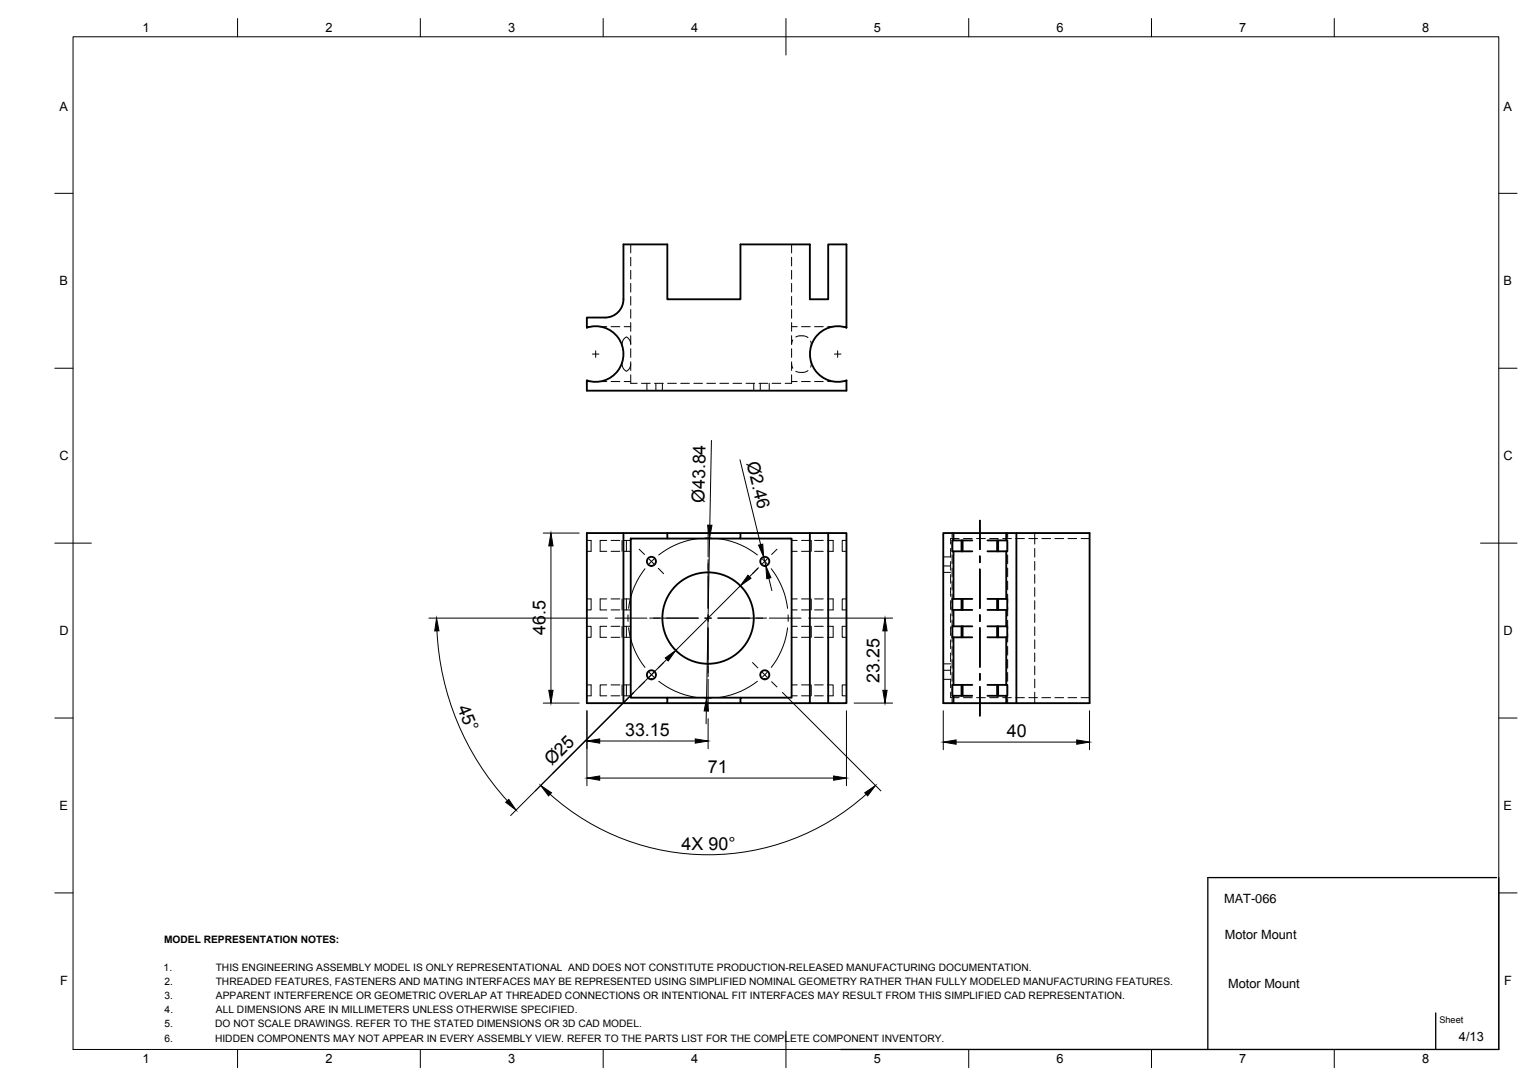
ISO-10303-21;
HEADER;
/* Generated by software containing ST-Developer
 * from STEP Tools, Inc. (www.steptools.com) 
 */

FILE_DESCRIPTION(
/* description */ ('CAx-IF Rec.Pracs.---Representation and Presentation of Product Manufa
cturing Information (PMI)---4.0---2014-10-13'),
/* implementation_level */ '2;1');

FILE_NAME(
/* name */ 'Motor Mount.step',
/* time_stamp */ '2026-10-24T15:58:00-07:00',
/* author */ (''),
/* organization */ (''),
/* preprocessor_version */ 'ST-DEVELOPER v20.2',
/* originating_system */ 'Autodesk Translation Framework v15.17.0.0',
/* authorisation */ '');

FILE_SCHEMA (('AP242_MANAGED_MODEL_BASED_3D_ENGINEERING_MIM_LF { 1 0 10303 442 2 1 4 }'));
ENDSEC;

DATA;
#10=MECHANICAL_DESIGN_GEOMETRIC_PRESENTATION_REPRESENTATION('',(#130),#8944);
#112=SHAPE_REPRESENTATION_RELATIONSHIP('SRR','None',#8994,#121);
#121=ADVANCED_BREP_SHAPE_REPRESENTATION('',(#139),#8935);
#130=STYLED_ITEM('',(#9053),#139);
#139=MANIFOLD_SOLID_BREP('Body1',#5151);
#165=CYLINDRICAL_SURFACE('',#5384,0.0125);
#166=CYLINDRICAL_SURFACE('',#5385,0.00123);
#167=CYLINDRICAL_SURFACE('',#5386,0.00123);
#168=CYLINDRICAL_SURFACE('',#5387,0.00123);
#169=CYLINDRICAL_SURFACE('',#5388,0.00123);
#170=CYLINDRICAL_SURFACE('',#5414,0.0076);
#171=CYLINDRICAL_SURFACE('',#5487,0.0023);
#172=CYLINDRICAL_SURFACE('',#5488,0.0023);
#173=CYLINDRICAL_SURFACE('',#5489,0.0023);
#174=CYLINDRICAL_SURFACE('',#5490,0.0023);
#175=CYLINDRICAL_SURFACE('',#5491,0.0023);
#176=CYLINDRICAL_SURFACE('',#5492,0.0023);
#177=CYLINDRICAL_SURFACE('',#5493,0.0023);
#178=CYLINDRICAL_SURFACE('',#5494,0.0023);
#179=CYLINDRICAL_SURFACE('',#5495,0.0023);
#180=CYLINDRICAL_SURFACE('',#5496,0.0023);
#181=CYLINDRICAL_SURFACE('',#5497,0.0023);
#182=CYLINDRICAL_SURFACE('',#5498,0.0023);
#183=CYLINDRICAL_SURFACE('',#5499,0.0023);
#184=CYLINDRICAL_SURFACE('',#5500,0.0023);
#185=CYLINDRICAL_SURFACE('',#5501,0.0023);
#186=CYLINDRICAL_SURFACE('',#5502,0.0023);
#187=CYLINDRICAL_SURFACE('',#5525,0.0076);
#188=CYLINDRICAL_SURFACE('',#5606,0.0023);
#189=CYLINDRICAL_SURFACE('',#5607,0.0023);
#190=CYLINDRICAL_SURFACE('',#5608,0.0023);
#191=CYLINDRICAL_SURFACE('',#5609,0.0023);
#192=CYLINDRICAL_SURFACE('',#5610,0.0023);
#193=CYLINDRICAL_SURFACE('',#5611,0.0023);
#194=CYLINDRICAL_SURFACE('',#5612,0.0023);
#195=CYLINDRICAL_SURFACE('',#5613,0.0023);
#196=CYLINDRICAL_SURFACE('',#5614,0.0023);
#197=CYLINDRICAL_SURFACE('',#5615,0.0023);
#198=CYLINDRICAL_SURFACE('',#5616,0.0023);
#199=CYLINDRICAL_SURFACE('',#5617,0.0023);
#200=CYLINDRICAL_SURFACE('',#5618,0.0023);
#201=CYLINDRICAL_SURFACE('',#5619,0.0023);
#202=CYLINDRICAL_SURFACE('',#5620,0.0023);
#203=CYLINDRICAL_SURFACE('',#5621,0.0023);
#204=CYLINDRICAL_SURFACE('',#5622,0.005);
#242=FACE_BOUND('',#613,.T.);
#243=FACE_BOUND('',#614,.T.);
#244=FACE_BOUND('',#615,.T.);
#245=FACE_BOUND('',#616,.T.);
#246=FACE_BOUND('',#617,.T.);
#247=FACE_BOUND('',#618,.T.);
#248=FACE_BOUND('',#619,.T.);
#249=FACE_BOUND('',#620,.T.);
#250=FACE_BOUND('',#634,.T.);
#251=FACE_BOUND('',#635,.T.);
#252=FACE_BOUND('',#636,.T.);
#253=FACE_BOUND('',#637,.T.);
#254=FACE_BOUND('',#638,.T.);
#255=FACE_BOUND('',#639,.T.);
#256=FACE_BOUND('',#640,.T.);
#257=FACE_BOUND('',#641,.T.);
#258=FACE_BOUND('',#659,.T.);
#259=FACE_BOUND('',#660,.T.);
#260=FACE_BOUND('',#661,.T.);
#261=FACE_BOUND('',#662,.T.);
#262=FACE_BOUND('',#663,.T.);
#263=FACE_BOUND('',#666,.T.);
#264=FACE_BOUND('',#667,.T.);
#265=FACE_BOUND('',#668,.T.);
#266=FACE_BOUND('',#669,.T.);
#267=FACE_BOUND('',#670,.T.);
#268=FACE_BOUND('',#694,.T.);
#269=FACE_BOUND('',#695,.T.);
#270=FACE_BOUND('',#696,.T.);
#271=FACE_BOUND('',#697,.T.);
#272=FACE_BOUND('',#698,.T.);
#273=FACE_BOUND('',#699,.T.);
#274=FACE_BOUND('',#700,.T.);
#275=FACE_BOUND('',#701,.T.);
#276=FACE_BOUND('',#758,.T.);
#277=FACE_BOUND('',#759,.T.);
#278=FACE_BOUND('',#760,.T.);
#279=FACE_BOUND('',#761,.T.);
#280=FACE_BOUND('',#762,.T.);
#281=FACE_BOUND('',#763,.T.);
#282=FACE_BOUND('',#764,.T.);
#283=FACE_BOUND('',#765,.T.);
#330=FACE_OUTER_BOUND('',#603,.T.);
#331=FACE_OUTER_BOUND('',#604,.T.);
#332=FACE_OUTER_BOUND('',#605,.T.);
#333=FACE_OUTER_BOUND('',#606,.T.);
#334=FACE_OUTER_BOUND('',#607,.T.);
#335=FACE_OUTER_BOUND('',#608,.T.);
#336=FACE_OUTER_BOUND('',#609,.T.);
#337=FACE_OUTER_BOUND('',#610,.T.);
#338=FACE_OUTER_BOUND('',#611,.T.);
#339=FACE_OUTER_BOUND('',#612,.T.);
#340=FACE_OUTER_BOUND('',#621,.T.);
#341=FACE_OUTER_BOUND('',#622,.T.);
#342=FACE_OUTER_BOUND('',#623,.T.);
#343=FACE_OUTER_BOUND('',#624,.T.);
#344=FACE_OUTER_BOUND('',#625,.T.);
#345=FACE_OUTER_BOUND('',#626,.T.);
#346=FACE_OUTER_BOUND('',#627,.T.);
#347=FACE_OUTER_BOUND('',#628,.T.);
#348=FACE_OUTER_BOUND('',#629,.T.);
#349=FACE_OUTER_BOUND('',#630,.T.);
#350=FACE_OUTER_BOUND('',#631,.T.);
#351=FACE_OUTER_BOUND('',#632,.T.);
#352=FACE_OUTER_BOUND('',#633,.T.);
#353=FACE_OUTER_BOUND('',#642,.T.);
#354=FACE_OUTER_BOUND('',#643,.T.);
#355=FACE_OUTER_BOUND('',#644,.T.);
#356=FACE_OUTER_BOUND('',#645,.T.);
#357=FACE_OUTER_BOUND('',#646,.T.);
#358=FACE_OUTER_BOUND('',#647,.T.);
#359=FACE_OUTER_BOUND('',#648,.T.);
#360=FACE_OUTER_BOUND('',#649,.T.);
#361=FACE_OUTER_BOUND('',#650,.T.);
#362=FACE_OUTER_BOUND('',#651,.T.);
#363=FACE_OUTER_BOUND('',#652,.T.);
#364=FACE_OUTER_BOUND('',#653,.T.);
#365=FACE_OUTER_BOUND('',#654,.T.);
#366=FACE_OUTER_BOUND('',#655,.T.);
#367=FACE_OUTER_BOUND('',#656,.T.);
#368=FACE_OUTER_BOUND('',#657,.T.);
#369=FACE_OUTER_BOUND('',#658,.T.);
#370=FACE_OUTER_BOUND('',#664,.T.);
#371=FACE_OUTER_BOUND('',#665,.T.);
#372=FACE_OUTER_BOUND('',#671,.T.);
#373=FACE_OUTER_BOUND('',#672,.T.);
#374=FACE_OUTER_BOUND('',#673,.T.);
#375=FACE_OUTER_BOUND('',#674,.T.);
#376=FACE_OUTER_BOUND('',#675,.T.);
#377=FACE_OUTER_BOUND('',#676,.T.);
#378=FACE_OUTER_BOUND('',#677,.T.);
#379=FACE_OUTER_BOUND('',#678,.T.);
#380=FACE_OUTER_BOUND('',#679,.T.);
#381=FACE_OUTER_BOUND('',#680,.T.);
#382=FACE_OUTER_BOUND('',#681,.T.);
#383=FACE_OUTER_BOUND('',#682,.T.);
#384=FACE_OUTER_BOUND('',#683,.T.);
#385=FACE_OUTER_BOUND('',#684,.T.);
#386=FACE_OUTER_BOUND('',#685,.T.);
#387=FACE_OUTER_BOUND('',#686,.T.);
#388=FACE_OUTER_BOUND('',#687,.T.);
#389=FACE_OUTER_BOUND('',#688,.T.);
#390=FACE_OUTER_BOUND('',#689,.T.);
#391=FACE_OUTER_BOUND('',#690,.T.);
#392=FACE_OUTER_BOUND('',#691,.T.);
#393=FACE_OUTER_BOUND('',#692,.T.);
#394=FACE_OUTER_BOUND('',#693,.T.);
#395=FACE_OUTER_BOUND('',#702,.T.);
#396=FACE_OUTER_BOUND('',#703,.T.);
#397=FACE_OUTER_BOUND('',#704,.T.);
#398=FACE_OUTER_BOUND('',#705,.T.);
#399=FACE_OUTER_BOUND('',#706,.T.);
#400=FACE_OUTER_BOUND('',#707,.T.);
#401=FACE_OUTER_BOUND('',#708,.T.);
#402=FACE_OUTER_BOUND('',#709,.T.);
#403=FACE_OUTER_BOUND('',#710,.T.);
#404=FACE_OUTER_BOUND('',#711,.T.);
#405=FACE_OUTER_BOUND('',#712,.T.);
#406=FACE_OUTER_BOUND('',#713,.T.);
#407=FACE_OUTER_BOUND('',#714,.T.);
#408=FACE_OUTER_BOUND('',#715,.T.);
#409=FACE_OUTER_BOUND('',#716,.T.);
#410=FACE_OUTER_BOUND('',#717,.T.);
#411=FACE_OUTER_BOUND('',#718,.T.);
#412=FACE_OUTER_BOUND('',#719,.T.);
#413=FACE_OUTER_BOUND('',#720,.T.);
#414=FACE_OUTER_BOUND('',#721,.T.);
#415=FACE_OUTER_BOUND('',#722,.T.);
#416=FACE_OUTER_BOUND('',#723,.T.);
#417=FACE_OUTER_BOUND('',#724,.T.);
#418=FACE_OUTER_BOUND('',#725,.T.);
#419=FACE_OUTER_BOUND('',#726,.T.);
#420=FACE_OUTER_BOUND('',#727,.T.);
#421=FACE_OUTER_BOUND('',#728,.T.);
#422=FACE_OUTER_BOUND('',#729,.T.);
#423=FACE_OUTER_BOUND('',#730,.T.);
#424=FACE_OUTER_BOUND('',#731,.T.);
#425=FACE_OUTER_BOUND('',#732,.T.);
#426=FACE_OUTER_BOUND('',#733,.T.);
#427=FACE_OUTER_BOUND('',#734,.T.);
#428=FACE_OUTER_BOUND('',#735,.T.);
#429=FACE_OUTER_BOUND('',#736,.T.);
#430=FACE_OUTER_BOUND('',#737,.T.);
#431=FACE_OUTER_BOUND('',#738,.T.);
#432=FACE_OUTER_BOUND('',#739,.T.);
#433=FACE_OUTER_BOUND('',#740,.T.);
#434=FACE_OUTER_BOUND('',#741,.T.);
#435=FACE_OUTER_BOUND('',#742,.T.);
#436=FACE_OUTER_BOUND('',#743,.T.);
#437=FACE_OUTER_BOUND('',#744,.T.);
#438=FACE_OUTER_BOUND('',#745,.T.);
#439=FACE_OUTER_BOUND('',#746,.T.);
#440=FACE_OUTER_BOUND('',#747,.T.);
#441=FACE_OUTER_BOUND('',#748,.T.);
#442=FACE_OUTER_BOUND('',#749,.T.);
#443=FACE_OUTER_BOUND('',#750,.T.);
#444=FACE_OUTER_BOUND('',#751,.T.);
#445=FACE_OUTER_BOUND('',#752,.T.);
#446=FACE_OUTER_BOUND('',#753,.T.);
#447=FACE_OUTER_BOUND('',#754,.T.);
#448=FACE_OUTER_BOUND('',#755,.T.);
#449=FACE_OUTER_BOUND('',#756,.T.);
#450=FACE_OUTER_BOUND('',#757,.T.);
#451=FACE_OUTER_BOUND('',#766,.T.);
#452=FACE_OUTER_BOUND('',#767,.T.);
#453=FACE_OUTER_BOUND('',#768,.T.);
#454=FACE_OUTER_BOUND('',#769,.T.);
#455=FACE_OUTER_BOUND('',#770,.T.);
#456=FACE_OUTER_BOUND('',#771,.T.);
#457=FACE_OUTER_BOUND('',#772,.T.);
#458=FACE_OUTER_BOUND('',#773,.T.);
#459=FACE_OUTER_BOUND('',#774,.T.);
#460=FACE_OUTER_BOUND('',#775,.T.);
#461=FACE_OUTER_BOUND('',#776,.T.);
#462=FACE_OUTER_BOUND('',#777,.T.);
#463=FACE_OUTER_BOUND('',#778,.T.);
#464=FACE_OUTER_BOUND('',#779,.T.);
#465=FACE_OUTER_BOUND('',#780,.T.);
#466=FACE_OUTER_BOUND('',#781,.T.);
#467=FACE_OUTER_BOUND('',#782,.T.);
#468=FACE_OUTER_BOUND('',#783,.T.);
#469=FACE_OUTER_BOUND('',#784,.T.);
#470=FACE_OUTER_BOUND('',#785,.T.);
#471=FACE_OUTER_BOUND('',#786,.T.);
#472=FACE_OUTER_BOUND('',#787,.T.);
#473=FACE_OUTER_BOUND('',#788,.T.);
#474=FACE_OUTER_BOUND('',#789,.T.);
#475=FACE_OUTER_BOUND('',#790,.T.);
#476=FACE_OUTER_BOUND('',#791,.T.);
#477=FACE_OUTER_BOUND('',#792,.T.);
#478=FACE_OUTER_BOUND('',#793,.T.);
#479=FACE_OUTER_BOUND('',#794,.T.);
#480=FACE_OUTER_BOUND('',#795,.T.);
#481=FACE_OUTER_BOUND('',#796,.T.);
#482=FACE_OUTER_BOUND('',#797,.T.);
#483=FACE_OUTER_BOUND('',#798,.T.);
#484=FACE_OUTER_BOUND('',#799,.T.);
#485=FACE_OUTER_BOUND('',#800,.T.);
#486=FACE_OUTER_BOUND('',#801,.T.);
#487=FACE_OUTER_BOUND('',#802,.T.);
#488=FACE_OUTER_BOUND('',#803,.T.);
#489=FACE_OUTER_BOUND('',#804,.T.);
#490=FACE_OUTER_BOUND('',#805,.T.);
#491=FACE_OUTER_BOUND('',#806,.T.);
#492=FACE_OUTER_BOUND('',#807,.T.);
#493=FACE_OUTER_BOUND('',#808,.T.);
#494=FACE_OUTER_BOUND('',#809,.T.);
#495=FACE_OUTER_BOUND('',#810,.T.);
#496=FACE_OUTER_BOUND('',#811,.T.);
#497=FACE_OUTER_BOUND('',#812,.T.);
#498=FACE_OUTER_BOUND('',#813,.T.);
#499=FACE_OUTER_BOUND('',#814,.T.);
#603=EDGE_LOOP('',(#3395,#3396,#3397,#3398));
#604=EDGE_LOOP('',(#3399,#3400,#3401,#3402));
#605=EDGE_LOOP('',(#3403,#3404,#3405,#3406));
#606=EDGE_LOOP('',(#3407,#3408,#3409,#3410,#3411,#3412,#3413,#3414));
#607=EDGE_LOOP('',(#3415,#3416,#3417,#3418,#3419,#3420,#3421,#3422));
#608=EDGE_LOOP('',(#3423,#3424,#3425,#3426,#3427,#3428,#3429,#3430));
#609=EDGE_LOOP('',(#3431,#3432,#3433,#3434));
#610=EDGE_LOOP('',(#3435,#3436,#3437,#3438));
#611=EDGE_LOOP('',(#3439,#3440,#3441,#3442));
#612=EDGE_LOOP('',(#3443,#3444,#3445,#3446));
#613=EDGE_LOOP('',(#3447,#3448,#3449,#3450));
#614=EDGE_LOOP('',(#3451,#3452,#3453,#3454));
#615=EDGE_LOOP('',(#3455,#3456,#3457,#3458));
#616=EDGE_LOOP('',(#3459,#3460,#3461,#3462));
#617=EDGE_LOOP('',(#3463,#3464,#3465,#3466));
#618=EDGE_LOOP('',(#3467,#3468,#3469,#3470));
#619=EDGE_LOOP('',(#3471,#3472,#3473,#3474));
#620=EDGE_LOOP('',(#3475,#3476,#3477,#3478));
#621=EDGE_LOOP('',(#3479,#3480,#3481));
#622=EDGE_LOOP('',(#3482,#3483,#3484));
#623=EDGE_LOOP('',(#3485,#3486,#3487));
#624=EDGE_LOOP('',(#3488,#3489,#3490));
#625=EDGE_LOOP('',(#3491,#3492,#3493));
#626=EDGE_LOOP('',(#3494,#3495,#3496));
#627=EDGE_LOOP('',(#3497,#3498,#3499,#3500));
#628=EDGE_LOOP('',(#3501,#3502,#3503));
#629=EDGE_LOOP('',(#3504,#3505,#3506));
#630=EDGE_LOOP('',(#3507,#3508,#3509));
#631=EDGE_LOOP('',(#3510,#3511,#3512,#3513,#3514,#3515,#3516,#3517,#3518,
#3519,#3520,#3521,#3522,#3523,#3524,#3525,#3526,#3527,#3528,#3529));
#632=EDGE_LOOP('',(#3530,#3531,#3532,#3533));
#633=EDGE_LOOP('',(#3534,#3535,#3536,#3537));
#634=EDGE_LOOP('',(#3538,#3539,#3540,#3541));
#635=EDGE_LOOP('',(#3542,#3543,#3544,#3545));
#636=EDGE_LOOP('',(#3546,#3547,#3548,#3549));
#637=EDGE_LOOP('',(#3550,#3551,#3552,#3553));
#638=EDGE_LOOP('',(#3554,#3555,#3556,#3557));
#639=EDGE_LOOP('',(#3558,#3559,#3560,#3561));
#640=EDGE_LOOP('',(#3562,#3563,#3564,#3565));
#641=EDGE_LOOP('',(#3566,#3567,#3568,#3569));
#642=EDGE_LOOP('',(#3570,#3571,#3572));
#643=EDGE_LOOP('',(#3573,#3574,#3575));
#644=EDGE_LOOP('',(#3576,#3577,#3578));
#645=EDGE_LOOP('',(#3579,#3580,#3581,#3582));
#646=EDGE_LOOP('',(#3583,#3584,#3585,#3586));
#647=EDGE_LOOP('',(#3587,#3588,#3589,#3590));
#648=EDGE_LOOP('',(#3591,#3592,#3593));
#649=EDGE_LOOP('',(#3594,#3595,#3596));
#650=EDGE_LOOP('',(#3597,#3598,#3599,#3600));
#651=EDGE_LOOP('',(#3601,#3602,#3603,#3604));
#652=EDGE_LOOP('',(#3605,#3606,#3607,#3608));
#653=EDGE_LOOP('',(#3609,#3610,#3611,#3612));
#654=EDGE_LOOP('',(#3613,#3614,#3615,#3616,#3617,#3618,#3619,#3620,#3621,
#3622,#3623,#3624,#3625,#3626,#3627,#3628,#3629,#3630,#3631,#3632));
#655=EDGE_LOOP('',(#3633,#3634,#3635,#3636));
#656=EDGE_LOOP('',(#3637,#3638,#3639,#3640,#3641,#3642,#3643,#3644));
#657=EDGE_LOOP('',(#3645,#3646,#3647,#3648,#3649,#3650,#3651,#3652,#3653,
#3654,#3655,#3656,#3657,#3658,#3659,#3660,#3661,#3662,#3663));
#658=EDGE_LOOP('',(#3664,#3665,#3666,#3667));
#659=EDGE_LOOP('',(#3668));
#660=EDGE_LOOP('',(#3669));
#661=EDGE_LOOP('',(#3670));
#662=EDGE_LOOP('',(#3671));
#663=EDGE_LOOP('',(#3672));
#664=EDGE_LOOP('',(#3673,#3674,#3675,#3676,#3677,#3678,#3679,#3680,#3681,
#3682,#3683,#3684,#3685,#3686,#3687,#3688,#3689,#3690,#3691));
#665=EDGE_LOOP('',(#3692,#3693,#3694,#3695));
#666=EDGE_LOOP('',(#3696));
#667=EDGE_LOOP('',(#3697));
#668=EDGE_LOOP('',(#3698));
#669=EDGE_LOOP('',(#3699));
#670=EDGE_LOOP('',(#3700));
#671=EDGE_LOOP('',(#3701,#3702,#3703,#3704));
#672=EDGE_LOOP('',(#3705,#3706,#3707,#3708));
#673=EDGE_LOOP('',(#3709,#3710,#3711,#3712));
#674=EDGE_LOOP('',(#3713,#3714,#3715,#3716));
#675=EDGE_LOOP('',(#3717,#3718,#3719,#3720));
#676=EDGE_LOOP('',(#3721,#3722,#3723,#3724));
#677=EDGE_LOOP('',(#3725,#3726,#3727,#3728));
#678=EDGE_LOOP('',(#3729,#3730,#3731,#3732));
#679=EDGE_LOOP('',(#3733,#3734,#3735,#3736));
#680=EDGE_LOOP('',(#3737,#3738,#3739));
#681=EDGE_LOOP('',(#3740,#3741,#3742));
#682=EDGE_LOOP('',(#3743,#3744,#3745));
#683=EDGE_LOOP('',(#3746,#3747,#3748));
#684=EDGE_LOOP('',(#3749,#3750,#3751));
#685=EDGE_LOOP('',(#3752,#3753,#3754));
#686=EDGE_LOOP('',(#3755,#3756,#3757,#3758));
#687=EDGE_LOOP('',(#3759,#3760,#3761));
#688=EDGE_LOOP('',(#3762,#3763,#3764));
#689=EDGE_LOOP('',(#3765,#3766,#3767));
#690=EDGE_LOOP('',(#3768,#3769,#3770));
#691=EDGE_LOOP('',(#3771,#3772,#3773));
#692=EDGE_LOOP('',(#3774,#3775,#3776,#3777,#3778,#3779,#3780,#3781,#3782,
#3783,#3784,#3785,#3786,#3787,#3788,#3789,#3790,#3791,#3792,#3793));
#693=EDGE_LOOP('',(#3794,#3795,#3796,#3797,#3798,#3799,#3800,#3801,#3802,
#3803,#3804,#3805,#3806,#3807,#3808,#3809,#3810,#3811,#3812,#3813,#3814,
#3815,#3816,#3817,#3818,#3819,#3820,#3821,#3822,#3823,#3824,#3825,#3826,
#3827,#3828,#3829));
#694=EDGE_LOOP('',(#3830,#3831,#3832,#3833));
#695=EDGE_LOOP('',(#3834,#3835,#3836,#3837));
#696=EDGE_LOOP('',(#3838,#3839,#3840,#3841));
#697=EDGE_LOOP('',(#3842,#3843,#3844,#3845));
#698=EDGE_LOOP('',(#3846,#3847,#3848,#3849));
#699=EDGE_LOOP('',(#3850,#3851,#3852,#3853));
#700=EDGE_LOOP('',(#3854,#3855,#3856,#3857));
#701=EDGE_LOOP('',(#3858,#3859,#3860,#3861));
#702=EDGE_LOOP('',(#3862,#3863,#3864,#3865,#3866));
#703=EDGE_LOOP('',(#3867,#3868,#3869,#3870));
#704=EDGE_LOOP('',(#3871,#3872,#3873,#3874,#3875));
#705=EDGE_LOOP('',(#3876,#3877,#3878,#3879));
#706=EDGE_LOOP('',(#3880,#3881,#3882,#3883,#3884));
#707=EDGE_LOOP('',(#3885,#3886,#3887,#3888,#3889));
#708=EDGE_LOOP('',(#3890,#3891,#3892,#3893,#3894));
#709=EDGE_LOOP('',(#3895,#3896,#3897,#3898));
#710=EDGE_LOOP('',(#3899,#3900,#3901,#3902,#3903));
#711=EDGE_LOOP('',(#3904,#3905,#3906,#3907,#3908));
#712=EDGE_LOOP('',(#3909,#3910,#3911,#3912));
#713=EDGE_LOOP('',(#3913,#3914,#3915,#3916,#3917));
#714=EDGE_LOOP('',(#3918,#3919,#3920,#3921,#3922));
#715=EDGE_LOOP('',(#3923,#3924,#3925,#3926));
#716=EDGE_LOOP('',(#3927,#3928,#3929,#3930,#3931));
#717=EDGE_LOOP('',(#3932,#3933,#3934,#3935,#3936));
#718=EDGE_LOOP('',(#3937,#3938,#3939,#3940));
#719=EDGE_LOOP('',(#3941,#3942,#3943,#3944,#3945));
#720=EDGE_LOOP('',(#3946,#3947,#3948,#3949));
#721=EDGE_LOOP('',(#3950,#3951,#3952,#3953,#3954));
#722=EDGE_LOOP('',(#3955,#3956,#3957,#3958,#3959));
#723=EDGE_LOOP('',(#3960,#3961,#3962,#3963));
#724=EDGE_LOOP('',(#3964,#3965,#3966,#3967,#3968));
#725=EDGE_LOOP('',(#3969,#3970,#3971,#3972,#3973));
#726=EDGE_LOOP('',(#3974,#3975,#3976,#3977));
#727=EDGE_LOOP('',(#3978,#3979,#3980,#3981));
#728=EDGE_LOOP('',(#3982,#3983,#3984,#3985));
#729=EDGE_LOOP('',(#3986,#3987,#3988,#3989));
#730=EDGE_LOOP('',(#3990,#3991,#3992,#3993));
#731=EDGE_LOOP('',(#3994,#3995,#3996,#3997));
#732=EDGE_LOOP('',(#3998,#3999,#4000,#4001));
#733=EDGE_LOOP('',(#4002,#4003,#4004,#4005));
#734=EDGE_LOOP('',(#4006,#4007,#4008,#4009));
#735=EDGE_LOOP('',(#4010,#4011,#4012,#4013));
#736=EDGE_LOOP('',(#4014,#4015,#4016,#4017));
#737=EDGE_LOOP('',(#4018,#4019,#4020,#4021));
#738=EDGE_LOOP('',(#4022,#4023,#4024,#4025));
#739=EDGE_LOOP('',(#4026,#4027,#4028,#4029));
#740=EDGE_LOOP('',(#4030,#4031,#4032,#4033));
#741=EDGE_LOOP('',(#4034,#4035,#4036,#4037));
#742=EDGE_LOOP('',(#4038,#4039,#4040));
#743=EDGE_LOOP('',(#4041,#4042,#4043,#4044));
#744=EDGE_LOOP('',(#4045,#4046,#4047));
#745=EDGE_LOOP('',(#4048,#4049,#4050,#4051));
#746=EDGE_LOOP('',(#4052,#4053,#4054));
#747=EDGE_LOOP('',(#4055,#4056,#4057));
#748=EDGE_LOOP('',(#4058,#4059,#4060));
#749=EDGE_LOOP('',(#4061,#4062,#4063,#4064));
#750=EDGE_LOOP('',(#4065,#4066,#4067));
#751=EDGE_LOOP('',(#4068,#4069,#4070,#4071));
#752=EDGE_LOOP('',(#4072,#4073,#4074));
#753=EDGE_LOOP('',(#4075,#4076,#4077,#4078));
#754=EDGE_LOOP('',(#4079,#4080,#4081,#4082));
#755=EDGE_LOOP('',(#4083,#4084,#4085,#4086));
#756=EDGE_LOOP('',(#4087,#4088,#4089,#4090,#4091,#4092,#4093,#4094,#4095,
#4096,#4097,#4098,#4099,#4100,#4101,#4102,#4103,#4104,#4105,#4106));
#757=EDGE_LOOP('',(#4107,#4108,#4109,#4110,#4111,#4112,#4113,#4114,#4115,
#4116,#4117,#4118,#4119,#4120,#4121,#4122,#4123,#4124,#4125,#4126,#4127,
#4128,#4129,#4130,#4131,#4132,#4133,#4134,#4135,#4136,#4137,#4138,#4139,
#4140,#4141,#4142));
#758=EDGE_LOOP('',(#4143,#4144,#4145,#4146));
#759=EDGE_LOOP('',(#4147,#4148,#4149,#4150));
#760=EDGE_LOOP('',(#4151,#4152,#4153,#4154));
#761=EDGE_LOOP('',(#4155,#4156,#4157,#4158));
#762=EDGE_LOOP('',(#4159,#4160,#4161,#4162));
#763=EDGE_LOOP('',(#4163,#4164,#4165,#4166));
#764=EDGE_LOOP('',(#4167,#4168,#4169,#4170));
#765=EDGE_LOOP('',(#4171,#4172,#4173,#4174));
#766=EDGE_LOOP('',(#4175,#4176,#4177,#4178));
#767=EDGE_LOOP('',(#4179,#4180,#4181,#4182,#4183,#4184));
#768=EDGE_LOOP('',(#4185,#4186,#4187,#4188));
#769=EDGE_LOOP('',(#4189,#4190,#4191,#4192,#4193,#4194));
#770=EDGE_LOOP('',(#4195,#4196,#4197,#4198));
#771=EDGE_LOOP('',(#4199,#4200,#4201,#4202,#4203,#4204));
#772=EDGE_LOOP('',(#4205,#4206,#4207,#4208));
#773=EDGE_LOOP('',(#4209,#4210,#4211,#4212,#4213,#4214));
#774=EDGE_LOOP('',(#4215,#4216,#4217,#4218));
#775=EDGE_LOOP('',(#4219,#4220,#4221,#4222,#4223,#4224));
#776=EDGE_LOOP('',(#4225,#4226,#4227,#4228));
#777=EDGE_LOOP('',(#4229,#4230,#4231,#4232,#4233,#4234));
#778=EDGE_LOOP('',(#4235,#4236,#4237,#4238));
#779=EDGE_LOOP('',(#4239,#4240,#4241,#4242,#4243,#4244));
#780=EDGE_LOOP('',(#4245,#4246,#4247,#4248));
#781=EDGE_LOOP('',(#4249,#4250,#4251,#4252,#4253,#4254));
#782=EDGE_LOOP('',(#4255,#4256,#4257,#4258));
#783=EDGE_LOOP('',(#4259,#4260,#4261,#4262,#4263,#4264));
#784=EDGE_LOOP('',(#4265,#4266,#4267,#4268));
#785=EDGE_LOOP('',(#4269,#4270,#4271,#4272,#4273,#4274));
#786=EDGE_LOOP('',(#4275,#4276,#4277,#4278));
#787=EDGE_LOOP('',(#4279,#4280,#4281,#4282,#4283,#4284));
#788=EDGE_LOOP('',(#4285,#4286,#4287,#4288));
#789=EDGE_LOOP('',(#4289,#4290,#4291,#4292,#4293,#4294));
#790=EDGE_LOOP('',(#4295,#4296,#4297,#4298));
#791=EDGE_LOOP('',(#4299,#4300,#4301,#4302,#4303,#4304));
#792=EDGE_LOOP('',(#4305,#4306,#4307,#4308));
#793=EDGE_LOOP('',(#4309,#4310,#4311,#4312,#4313,#4314));
#794=EDGE_LOOP('',(#4315,#4316,#4317,#4318));
#795=EDGE_LOOP('',(#4319,#4320,#4321,#4322,#4323,#4324));
#796=EDGE_LOOP('',(#4325,#4326,#4327,#4328));
#797=EDGE_LOOP('',(#4329,#4330,#4331,#4332,#4333,#4334));
#798=EDGE_LOOP('',(#4335,#4336,#4337,#4338));
#799=EDGE_LOOP('',(#4339,#4340,#4341,#4342));
#800=EDGE_LOOP('',(#4343,#4344,#4345,#4346));
#801=EDGE_LOOP('',(#4347,#4348,#4349,#4350));
#802=EDGE_LOOP('',(#4351,#4352,#4353,#4354));
#803=EDGE_LOOP('',(#4355,#4356,#4357,#4358));
#804=EDGE_LOOP('',(#4359,#4360,#4361,#4362));
#805=EDGE_LOOP('',(#4363,#4364,#4365,#4366));
#806=EDGE_LOOP('',(#4367,#4368,#4369,#4370));
#807=EDGE_LOOP('',(#4371,#4372,#4373,#4374));
#808=EDGE_LOOP('',(#4375,#4376,#4377,#4378));
#809=EDGE_LOOP('',(#4379,#4380,#4381,#4382));
#810=EDGE_LOOP('',(#4383,#4384,#4385,#4386));
#811=EDGE_LOOP('',(#4387,#4388,#4389,#4390));
#812=EDGE_LOOP('',(#4391,#4392,#4393,#4394));
#813=EDGE_LOOP('',(#4395,#4396,#4397,#4398));
#814=EDGE_LOOP('',(#4399,#4400,#4401,#4402));
#941=CIRCLE('',#5320,0.0076);
#942=CIRCLE('',#5322,0.0076);
#943=CIRCLE('',#5324,0.0076);
#944=CIRCLE('',#5326,0.0076);
#945=CIRCLE('',#5328,0.0076);
#946=CIRCLE('',#5330,0.0076);
#947=CIRCLE('',#5333,0.0076);
#948=CIRCLE('',#5335,0.0076);
#949=CIRCLE('',#5337,0.0076);
#950=CIRCLE('',#5342,0.0076);
#951=CIRCLE('',#5344,0.0076);
#952=CIRCLE('',#5346,0.0076);
#953=CIRCLE('',#5351,0.0076);
#954=CIRCLE('',#5353,0.0076);
#955=CIRCLE('',#5362,0.0076);
#956=CIRCLE('',#5363,0.005);
#957=CIRCLE('',#5364,0.0076);
#958=CIRCLE('',#5366,0.00123);
#959=CIRCLE('',#5367,0.00123);
#960=CIRCLE('',#5368,0.00123);
#961=CIRCLE('',#5369,0.00123);
#962=CIRCLE('',#5370,0.0125);
#963=CIRCLE('',#5372,0.0076);
#964=CIRCLE('',#5373,0.0076);
#965=CIRCLE('',#5374,0.005);
#966=CIRCLE('',#5376,0.00123);
#967=CIRCLE('',#5377,0.00123);
#968=CIRCLE('',#5378,0.00123);
#969=CIRCLE('',#5379,0.00123);
#970=CIRCLE('',#5380,0.0125);
#971=CIRCLE('',#5391,0.0076);
#972=CIRCLE('',#5393,0.0076);
#973=CIRCLE('',#5395,0.0076);
#974=CIRCLE('',#5397,0.0076);
#975=CIRCLE('',#5399,0.0076);
#976=CIRCLE('',#5401,0.0076);
#977=CIRCLE('',#5404,0.0076);
#978=CIRCLE('',#5406,0.0076);
#979=CIRCLE('',#5408,0.0076);
#980=CIRCLE('',#5410,0.0076);
#981=CIRCLE('',#5412,0.0076);
#982=CIRCLE('',#5415,0.0076);
#983=CIRCLE('',#5416,0.0076);
#984=CIRCLE('',#5417,0.0076);
#985=CIRCLE('',#5418,0.0076);
#986=CIRCLE('',#5419,0.0076);
#987=CIRCLE('',#5420,0.0076);
#988=CIRCLE('',#5421,0.0076);
#989=CIRCLE('',#5422,0.0076);
#990=CIRCLE('',#5423,0.0076);
#991=CIRCLE('',#5424,0.0076);
#992=CIRCLE('',#5425,0.0076);
#993=CIRCLE('',#5426,0.0076);
#994=CIRCLE('',#5427,0.0076);
#995=CIRCLE('',#5428,0.0076);
#996=CIRCLE('',#5429,0.0076);
#997=CIRCLE('',#5430,0.0076);
#998=CIRCLE('',#5432,0.0023);
#999=CIRCLE('',#5433,0.0023);
#1000=CIRCLE('',#5436,0.0023);
#1001=CIRCLE('',#5437,0.0023);
#1002=CIRCLE('',#5440,0.0023);
#1003=CIRCLE('',#5441,0.0023);
#1004=CIRCLE('',#5443,0.0023);
#1005=CIRCLE('',#5444,0.0023);
#1006=CIRCLE('',#5446,0.0023);
#1007=CIRCLE('',#5447,0.0023);
#1008=CIRCLE('',#5450,0.0023);
#1009=CIRCLE('',#5451,0.0023);
#1010=CIRCLE('',#5453,0.0023);
#1011=CIRCLE('',#5454,0.0023);
#1012=CIRCLE('',#5457,0.0023);
#1013=CIRCLE('',#5458,0.0023);
#1014=CIRCLE('',#5460,0.0023);
#1015=CIRCLE('',#5461,0.0023);
#1016=CIRCLE('',#5464,0.0023);
#1017=CIRCLE('',#5465,0.0023);
#1018=CIRCLE('',#5467,0.0023);
#1019=CIRCLE('',#5468,0.0023);
#1020=CIRCLE('',#5471,0.0023);
#1021=CIRCLE('',#5472,0.0023);
#1022=CIRCLE('',#5475,0.0023);
#1023=CIRCLE('',#5476,0.0023);
#1024=CIRCLE('',#5478,0.0023);
#1025=CIRCLE('',#5479,0.0023);
#1026=CIRCLE('',#5482,0.0023);
#1027=CIRCLE('',#5483,0.0023);
#1028=CIRCLE('',#5485,0.0023);
#1029=CIRCLE('',#5486,0.0023);
#1030=CIRCLE('',#5504,0.0076);
#1031=CIRCLE('',#5507,0.0076);
#1032=CIRCLE('',#5510,0.0076);
#1033=CIRCLE('',#5512,0.0076);
#1034=CIRCLE('',#5514,0.0076);
#1035=CIRCLE('',#5517,0.0076);
#1036=CIRCLE('',#5520,0.0076);
#1037=CIRCLE('',#5526,0.0076);
#1038=CIRCLE('',#5527,0.0076);
#1039=CIRCLE('',#5528,0.0076);
#1040=CIRCLE('',#5529,0.0076);
#1041=CIRCLE('',#5530,0.0076);
#1042=CIRCLE('',#5531,0.0076);
#1043=CIRCLE('',#5532,0.0076);
#1044=CIRCLE('',#5533,0.0076);
#1045=CIRCLE('',#5534,0.0076);
#1046=CIRCLE('',#5535,0.0076);
#1047=CIRCLE('',#5536,0.0076);
#1048=CIRCLE('',#5537,0.0076);
#1049=CIRCLE('',#5538,0.0076);
#1050=CIRCLE('',#5539,0.0076);
#1051=CIRCLE('',#5540,0.0076);
#1052=CIRCLE('',#5541,0.0076);
#1053=CIRCLE('',#5544,0.0023);
#1054=CIRCLE('',#5545,0.0023);
#1055=CIRCLE('',#5548,0.0023);
#1056=CIRCLE('',#5549,0.0023);
#1057=CIRCLE('',#5552,0.0023);
#1058=CIRCLE('',#5553,0.0023);
#1059=CIRCLE('',#5556,0.0023);
#1060=CIRCLE('',#5557,0.0023);
#1061=CIRCLE('',#5560,0.0023);
#1062=CIRCLE('',#5561,0.0023);
#1063=CIRCLE('',#5564,0.0023);
#1064=CIRCLE('',#5565,0.0023);
#1065=CIRCLE('',#5568,0.0023);
#1066=CIRCLE('',#5569,0.0023);
#1067=CIRCLE('',#5572,0.0023);
#1068=CIRCLE('',#5573,0.0023);
#1069=CIRCLE('',#5576,0.0023);
#1070=CIRCLE('',#5577,0.0023);
#1071=CIRCLE('',#5580,0.0023);
#1072=CIRCLE('',#5581,0.0023);
#1073=CIRCLE('',#5584,0.0023);
#1074=CIRCLE('',#5585,0.0023);
#1075=CIRCLE('',#5588,0.0023);
#1076=CIRCLE('',#5589,0.0023);
#1077=CIRCLE('',#5592,0.0023);
#1078=CIRCLE('',#5593,0.0023);
#1079=CIRCLE('',#5596,0.0023);
#1080=CIRCLE('',#5597,0.0023);
#1081=CIRCLE('',#5600,0.0023);
#1082=CIRCLE('',#5601,0.0023);
#1083=CIRCLE('',#5604,0.0023);
#1084=CIRCLE('',#5605,0.0023);
#1204=LINE('',#7535,#1659);
#1205=LINE('',#7537,#1660);
#1206=LINE('',#7539,#1661);
#1207=LINE('',#7540,#1662);
#1208=LINE('',#7544,#1663);
#1209=LINE('',#7546,#1664);
#1210=LINE('',#7548,#1665);
#1211=LINE('',#7549,#1666);
#1212=LINE('',#7551,#1667);
#1213=LINE('',#7552,#1668);
#1214=LINE('',#7555,#1669);
#1215=LINE('',#7557,#1670);
#1216=LINE('',#7559,#1671);
#1217=LINE('',#7561,#1672);
#1218=LINE('',#7563,#1673);
#1219=LINE('',#7565,#1674);
#1220=LINE('',#7566,#1675);
#1221=LINE('',#7569,#1676);
#1222=LINE('',#7571,#1677);
#1223=LINE('',#7573,#1678);
#1224=LINE('',#7575,#1679);
#1225=LINE('',#7577,#1680);
#1226=LINE('',#7579,#1681);
#1227=LINE('',#7580,#1682);
#1228=LINE('',#7583,#1683);
#1229=LINE('',#7585,#1684);
#1230=LINE('',#7586,#1685);
#1231=LINE('',#7590,#1686);
#1232=LINE('',#7592,#1687);
#1233=LINE('',#7594,#1688);
#1234=LINE('',#7595,#1689);
#1235=LINE('',#7598,#1690);
#1236=LINE('',#7600,#1691);
#1237=LINE('',#7601,#1692);
#1238=LINE('',#7605,#1693);
#1239=LINE('',#7606,#1694);
#1240=LINE('',#7607,#1695);
#1241=LINE('',#7610,#1696);
#1242=LINE('',#7611,#1697);
#1243=LINE('',#7614,#1698);
#1244=LINE('',#7616,#1699);
#1245=LINE('',#7618,#1700);
#1246=LINE('',#7619,#1701);
#1247=LINE('',#7622,#1702);
#1248=LINE('',#7624,#1703);
#1249=LINE('',#7626,#1704);
#1250=LINE('',#7627,#1705);
#1251=LINE('',#7630,#1706);
#1252=LINE('',#7632,#1707);
#1253=LINE('',#7634,#1708);
#1254=LINE('',#7635,#1709);
#1255=LINE('',#7638,#1710);
#1256=LINE('',#7640,#1711);
#1257=LINE('',#7642,#1712);
#1258=LINE('',#7643,#1713);
#1259=LINE('',#7646,#1714);
#1260=LINE('',#7648,#1715);
#1261=LINE('',#7650,#1716);
#1262=LINE('',#7651,#1717);
#1263=LINE('',#7654,#1718);
#1264=LINE('',#7656,#1719);
#1265=LINE('',#7658,#1720);
#1266=LINE('',#7659,#1721);
#1267=LINE('',#7662,#1722);
#1268=LINE('',#7664,#1723);
#1269=LINE('',#7666,#1724);
#1270=LINE('',#7667,#1725);
#1271=LINE('',#7670,#1726);
#1272=LINE('',#7672,#1727);
#1273=LINE('',#7674,#1728);
#1274=LINE('',#7675,#1729);
#1275=LINE('',#7681,#1730);
#1276=LINE('',#7682,#1731);
#1277=LINE('',#7686,#1732);
#1278=LINE('',#7689,#1733);
#1279=LINE('',#7695,#1734);
#1280=LINE('',#7696,#1735);
#1281=LINE('',#7700,#1736);
#1282=LINE('',#7703,#1737);
#1283=LINE('',#7709,#1738);
#1284=LINE('',#7710,#1739);
#1285=LINE('',#7716,#1740);
#1286=LINE('',#7717,#1741);
#1287=LINE('',#7720,#1742);
#1288=LINE('',#7722,#1743);
#1289=LINE('',#7723,#1744);
#1290=LINE('',#7727,#1745);
#1291=LINE('',#7730,#1746);
#1292=LINE('',#7736,#1747);
#1293=LINE('',#7737,#1748);
#1294=LINE('',#7741,#1749);
#1295=LINE('',#7744,#1750);
#1296=LINE('',#7748,#1751);
#1297=LINE('',#7749,#1752);
#1298=LINE('',#7750,#1753);
#1299=LINE('',#7751,#1754);
#1300=LINE('',#7752,#1755);
#1301=LINE('',#7753,#1756);
#1302=LINE('',#7755,#1757);
#1303=LINE('',#7756,#1758);
#1304=LINE('',#7757,#1759);
#1305=LINE('',#7759,#1760);
#1306=LINE('',#7761,#1761);
#1307=LINE('',#7762,#1762);
#1308=LINE('',#7764,#1763);
#1309=LINE('',#7765,#1764);
#1310=LINE('',#7768,#1765);
#1311=LINE('',#7769,#1766);
#1312=LINE('',#7772,#1767);
#1313=LINE('',#7774,#1768);
#1314=LINE('',#7776,#1769);
#1315=LINE('',#7777,#1770);
#1316=LINE('',#7780,#1771);
#1317=LINE('',#7782,#1772);
#1318=LINE('',#7784,#1773);
#1319=LINE('',#7785,#1774);
#1320=LINE('',#7788,#1775);
#1321=LINE('',#7790,#1776);
#1322=LINE('',#7792,#1777);
#1323=LINE('',#7793,#1778);
#1324=LINE('',#7796,#1779);
#1325=LINE('',#7798,#1780);
#1326=LINE('',#7800,#1781);
#1327=LINE('',#7801,#1782);
#1328=LINE('',#7804,#1783);
#1329=LINE('',#7806,#1784);
#1330=LINE('',#7808,#1785);
#1331=LINE('',#7809,#1786);
#1332=LINE('',#7812,#1787);
#1333=LINE('',#7814,#1788);
#1334=LINE('',#7816,#1789);
#1335=LINE('',#7817,#1790);
#1336=LINE('',#7820,#1791);
#1337=LINE('',#7822,#1792);
#1338=LINE('',#7824,#1793);
#1339=LINE('',#7825,#1794);
#1340=LINE('',#7828,#1795);
#1341=LINE('',#7830,#1796);
#1342=LINE('',#7832,#1797);
#1343=LINE('',#7833,#1798);
#1344=LINE('',#7839,#1799);
#1345=LINE('',#7840,#1800);
#1346=LINE('',#7844,#1801);
#1347=LINE('',#7847,#1802);
#1348=LINE('',#7851,#1803);
#1349=LINE('',#7854,#1804);
#1350=LINE('',#7858,#1805);
#1351=LINE('',#7860,#1806);
#1352=LINE('',#7862,#1807);
#1353=LINE('',#7863,#1808);
#1354=LINE('',#7867,#1809);
#1355=LINE('',#7869,#1810);
#1356=LINE('',#7871,#1811);
#1357=LINE('',#7872,#1812);
#1358=LINE('',#7876,#1813);
#1359=LINE('',#7878,#1814);
#1360=LINE('',#7880,#1815);
#1361=LINE('',#7881,#1816);
#1362=LINE('',#7887,#1817);
#1363=LINE('',#7888,#1818);
#1364=LINE('',#7892,#1819);
#1365=LINE('',#7895,#1820);
#1366=LINE('',#7899,#1821);
#1367=LINE('',#7901,#1822);
#1368=LINE('',#7903,#1823);
#1369=LINE('',#7904,#1824);
#1370=LINE('',#7906,#1825);
#1371=LINE('',#7907,#1826);
#1372=LINE('',#7910,#1827);
#1373=LINE('',#7912,#1828);
#1374=LINE('',#7913,#1829);
#1375=LINE('',#7915,#1830);
#1376=LINE('',#7916,#1831);
#1377=LINE('',#7920,#1832);
#1378=LINE('',#7922,#1833);
#1379=LINE('',#7923,#1834);
#1380=LINE('',#7925,#1835);
#1381=LINE('',#7927,#1836);
#1382=LINE('',#7928,#1837);
#1383=LINE('',#7930,#1838);
#1384=LINE('',#7932,#1839);
#1385=LINE('',#7933,#1840);
#1386=LINE('',#7935,#1841);
#1387=LINE('',#7937,#1842);
#1388=LINE('',#7938,#1843);
#1389=LINE('',#7940,#1844);
#1390=LINE('',#7942,#1845);
#1391=LINE('',#7944,#1846);
#1392=LINE('',#7945,#1847);
#1393=LINE('',#7948,#1848);
#1394=LINE('',#7950,#1849);
#1395=LINE('',#7951,#1850);
#1396=LINE('',#7955,#1851);
#1397=LINE('',#7956,#1852);
#1398=LINE('',#7957,#1853);
#1399=LINE('',#7958,#1854);
#1400=LINE('',#7962,#1855);
#1401=LINE('',#7964,#1856);
#1402=LINE('',#7966,#1857);
#1403=LINE('',#7967,#1858);
#1404=LINE('',#7971,#1859);
#1405=LINE('',#7973,#1860);
#1406=LINE('',#7975,#1861);
#1407=LINE('',#7977,#1862);
#1408=LINE('',#7990,#1863);
#1409=LINE('',#7995,#1864);
#1410=LINE('',#7997,#1865);
#1411=LINE('',#8011,#1866);
#1412=LINE('',#8013,#1867);
#1413=LINE('',#8016,#1868);
#1414=LINE('',#8018,#1869);
#1415=LINE('',#8020,#1870);
#1416=LINE('',#8022,#1871);
#1417=LINE('',#8024,#1872);
#1418=LINE('',#8026,#1873);
#1419=LINE('',#8027,#1874);
#1420=LINE('',#8031,#1875);
#1421=LINE('',#8045,#1876);
#1422=LINE('',#8046,#1877);
#1423=LINE('',#8049,#1878);
#1424=LINE('',#8051,#1879);
#1425=LINE('',#8052,#1880);
#1426=LINE('',#8056,#1881);
#1427=LINE('',#8066,#1882);
#1428=LINE('',#8067,#1883);
#1429=LINE('',#8068,#1884);
#1430=LINE('',#8069,#1885);
#1431=LINE('',#8070,#1886);
#1432=LINE('',#8076,#1887);
#1433=LINE('',#8079,#1888);
#1434=LINE('',#8084,#1889);
#1435=LINE('',#8087,#1890);
#1436=LINE('',#8090,#1891);
#1437=LINE('',#8094,#1892);
#1438=LINE('',#8098,#1893);
#1439=LINE('',#8102,#1894);
#1440=LINE('',#8106,#1895);
#1441=LINE('',#8110,#1896);
#1442=LINE('',#8114,#1897);
#1443=LINE('',#8118,#1898);
#1444=LINE('',#8124,#1899);
#1445=LINE('',#8127,#1900);
#1446=LINE('',#8130,#1901);
#1447=LINE('',#8134,#1902);
#1448=LINE('',#8140,#1903);
#1449=LINE('',#8142,#1904);
#1450=LINE('',#8148,#1905);
#1451=LINE('',#8149,#1906);
#1452=LINE('',#8162,#1907);
#1453=LINE('',#8164,#1908);
#1454=LINE('',#8173,#1909);
#1455=LINE('',#8175,#1910);
#1456=LINE('',#8184,#1911);
#1457=LINE('',#8186,#1912);
#1458=LINE('',#8195,#1913);
#1459=LINE('',#8197,#1914);
#1460=LINE('',#8203,#1915);
#1461=LINE('',#8204,#1916);
#1462=LINE('',#8214,#1917);
#1463=LINE('',#8215,#1918);
#1464=LINE('',#8225,#1919);
#1465=LINE('',#8228,#1920);
#1466=LINE('',#8231,#1921);
#1467=LINE('',#8234,#1922);
#1468=LINE('',#8237,#1923);
#1469=LINE('',#8240,#1924);
#1470=LINE('',#8243,#1925);
#1471=LINE('',#8246,#1926);
#1472=LINE('',#8253,#1927);
#1473=LINE('',#8254,#1928);
#1474=LINE('',#8257,#1929);
#1475=LINE('',#8259,#1930);
#1476=LINE('',#8260,#1931);
#1477=LINE('',#8264,#1932);
#1478=LINE('',#8267,#1933);
#1479=LINE('',#8269,#1934);
#1480=LINE('',#8270,#1935);
#1481=LINE('',#8274,#1936);
#1482=LINE('',#8282,#1937);
#1483=LINE('',#8283,#1938);
#1484=LINE('',#8285,#1939);
#1485=LINE('',#8286,#1940);
#1486=LINE('',#8292,#1941);
#1487=LINE('',#8293,#1942);
#1488=LINE('',#8296,#1943);
#1489=LINE('',#8298,#1944);
#1490=LINE('',#8299,#1945);
#1491=LINE('',#8303,#1946);
#1492=LINE('',#8305,#1947);
#1493=LINE('',#8307,#1948);
#1494=LINE('',#8309,#1949);
#1495=LINE('',#8311,#1950);
#1496=LINE('',#8312,#1951);
#1497=LINE('',#8313,#1952);
#1498=LINE('',#8314,#1953);
#1499=LINE('',#8315,#1954);
#1500=LINE('',#8321,#1955);
#1501=LINE('',#8324,#1956);
#1502=LINE('',#8327,#1957);
#1503=LINE('',#8331,#1958);
#1504=LINE('',#8335,#1959);
#1505=LINE('',#8339,#1960);
#1506=LINE('',#8343,#1961);
#1507=LINE('',#8347,#1962);
#1508=LINE('',#8351,#1963);
#1509=LINE('',#8355,#1964);
#1510=LINE('',#8361,#1965);
#1511=LINE('',#8364,#1966);
#1512=LINE('',#8367,#1967);
#1513=LINE('',#8371,#1968);
#1514=LINE('',#8377,#1969);
#1515=LINE('',#8380,#1970);
#1516=LINE('',#8382,#1971);
#1517=LINE('',#8383,#1972);
#1518=LINE('',#8388,#1973);
#1519=LINE('',#8393,#1974);
#1520=LINE('',#8394,#1975);
#1521=LINE('',#8395,#1976);
#1522=LINE('',#8402,#1977);
#1523=LINE('',#8404,#1978);
#1524=LINE('',#8406,#1979);
#1525=LINE('',#8407,#1980);
#1526=LINE('',#8410,#1981);
#1527=LINE('',#8413,#1982);
#1528=LINE('',#8418,#1983);
#1529=LINE('',#8419,#1984);
#1530=LINE('',#8424,#1985);
#1531=LINE('',#8429,#1986);
#1532=LINE('',#8430,#1987);
#1533=LINE('',#8431,#1988);
#1534=LINE('',#8438,#1989);
#1535=LINE('',#8440,#1990);
#1536=LINE('',#8442,#1991);
#1537=LINE('',#8443,#1992);
#1538=LINE('',#8446,#1993);
#1539=LINE('',#8449,#1994);
#1540=LINE('',#8456,#1995);
#1541=LINE('',#8458,#1996);
#1542=LINE('',#8460,#1997);
#1543=LINE('',#8461,#1998);
#1544=LINE('',#8464,#1999);
#1545=LINE('',#8467,#2000);
#1546=LINE('',#8474,#2001);
#1547=LINE('',#8476,#2002);
#1548=LINE('',#8478,#2003);
#1549=LINE('',#8479,#2004);
#1550=LINE('',#8482,#2005);
#1551=LINE('',#8485,#2006);
#1552=LINE('',#8492,#2007);
#1553=LINE('',#8494,#2008);
#1554=LINE('',#8496,#2009);
#1555=LINE('',#8497,#2010);
#1556=LINE('',#8500,#2011);
#1557=LINE('',#8503,#2012);
#1558=LINE('',#8508,#2013);
#1559=LINE('',#8509,#2014);
#1560=LINE('',#8514,#2015);
#1561=LINE('',#8519,#2016);
#1562=LINE('',#8520,#2017);
#1563=LINE('',#8521,#2018);
#1659=VECTOR('',#5951,0.01);
#1660=VECTOR('',#5952,0.01);
#1661=VECTOR('',#5953,0.01);
#1662=VECTOR('',#5954,0.01);
#1663=VECTOR('',#5957,0.01);
#1664=VECTOR('',#5958,0.01);
#1665=VECTOR('',#5959,0.01);
#1666=VECTOR('',#5960,0.01);
#1667=VECTOR('',#5963,0.01);
#1668=VECTOR('',#5964,0.01);
#1669=VECTOR('',#5967,1.);
#1670=VECTOR('',#5968,1.);
#1671=VECTOR('',#5969,1.);
#1672=VECTOR('',#5970,1.);
#1673=VECTOR('',#5971,1.);
#1674=VECTOR('',#5972,1.);
#1675=VECTOR('',#5973,1.);
#1676=VECTOR('',#5976,1.);
#1677=VECTOR('',#5977,1.);
#1678=VECTOR('',#5978,1.);
#1679=VECTOR('',#5979,1.);
#1680=VECTOR('',#5980,1.);
#1681=VECTOR('',#5981,1.);
#1682=VECTOR('',#5982,1.);
#1683=VECTOR('',#5985,1.);
#1684=VECTOR('',#5986,1.);
#1685=VECTOR('',#5987,1.);
#1686=VECTOR('',#5990,0.01);
#1687=VECTOR('',#5991,0.01);
#1688=VECTOR('',#5992,0.01);
#1689=VECTOR('',#5993,1.);
#1690=VECTOR('',#5996,0.01);
#1691=VECTOR('',#5997,0.01);
#1692=VECTOR('',#5998,0.01);
#1693=VECTOR('',#6001,0.01);
#1694=VECTOR('',#6002,0.01);
#1695=VECTOR('',#6003,0.01);
#1696=VECTOR('',#6006,1.);
#1697=VECTOR('',#6007,1.);
#1698=VECTOR('',#6008,1.);
#1699=VECTOR('',#6009,1.);
#1700=VECTOR('',#6010,1.);
#1701=VECTOR('',#6011,1.);
#1702=VECTOR('',#6012,1.);
#1703=VECTOR('',#6013,1.);
#1704=VECTOR('',#6014,1.);
#1705=VECTOR('',#6015,1.);
#1706=VECTOR('',#6016,1.);
#1707=VECTOR('',#6017,1.);
#1708=VECTOR('',#6018,1.);
#1709=VECTOR('',#6019,1.);
#1710=VECTOR('',#6020,1.);
#1711=VECTOR('',#6021,1.);
#1712=VECTOR('',#6022,1.);
#1713=VECTOR('',#6023,1.);
#1714=VECTOR('',#6024,1.);
#1715=VECTOR('',#6025,1.);
#1716=VECTOR('',#6026,1.);
#1717=VECTOR('',#6027,1.);
#1718=VECTOR('',#6028,1.);
#1719=VECTOR('',#6029,1.);
#1720=VECTOR('',#6030,1.);
#1721=VECTOR('',#6031,1.);
#1722=VECTOR('',#6032,1.);
#1723=VECTOR('',#6033,1.);
#1724=VECTOR('',#6034,1.);
#1725=VECTOR('',#6035,1.);
#1726=VECTOR('',#6036,1.);
#1727=VECTOR('',#6037,1.);
#1728=VECTOR('',#6038,1.);
#1729=VECTOR('',#6039,1.);
#1730=VECTOR('',#6044,1.);
#1731=VECTOR('',#6045,1.);
#1732=VECTOR('',#6048,1.);
#1733=VECTOR('',#6051,1.);
#1734=VECTOR('',#6056,1.);
#1735=VECTOR('',#6057,1.);
#1736=VECTOR('',#6060,1.);
#1737=VECTOR('',#6063,1.);
#1738=VECTOR('',#6068,1.);
#1739=VECTOR('',#6069,1.);
#1740=VECTOR('',#6074,1.);
#1741=VECTOR('',#6075,1.);
#1742=VECTOR('',#6078,1.);
#1743=VECTOR('',#6079,1.);
#1744=VECTOR('',#6080,1.);
#1745=VECTOR('',#6083,1.);
#1746=VECTOR('',#6086,1.);
#1747=VECTOR('',#6091,1.);
#1748=VECTOR('',#6092,1.);
#1749=VECTOR('',#6095,1.);
#1750=VECTOR('',#6098,1.);
#1751=VECTOR('',#6101,1.);
#1752=VECTOR('',#6102,1.);
#1753=VECTOR('',#6103,1.);
#1754=VECTOR('',#6104,1.);
#1755=VECTOR('',#6105,1.);
#1756=VECTOR('',#6106,1.);
#1757=VECTOR('',#6107,1.);
#1758=VECTOR('',#6108,1.);
#1759=VECTOR('',#6109,1.);
#1760=VECTOR('',#6110,1.);
#1761=VECTOR('',#6111,1.);
#1762=VECTOR('',#6112,1.);
#1763=VECTOR('',#6115,1.);
#1764=VECTOR('',#6116,1.);
#1765=VECTOR('',#6119,1.);
#1766=VECTOR('',#6120,1.);
#1767=VECTOR('',#6121,1.);
#1768=VECTOR('',#6122,1.);
#1769=VECTOR('',#6123,1.);
#1770=VECTOR('',#6124,1.);
#1771=VECTOR('',#6125,1.);
#1772=VECTOR('',#6126,1.);
#1773=VECTOR('',#6127,1.);
#1774=VECTOR('',#6128,1.);
#1775=VECTOR('',#6129,1.);
#1776=VECTOR('',#6130,1.);
#1777=VECTOR('',#6131,1.);
#1778=VECTOR('',#6132,1.);
#1779=VECTOR('',#6133,1.);
#1780=VECTOR('',#6134,1.);
#1781=VECTOR('',#6135,1.);
#1782=VECTOR('',#6136,1.);
#1783=VECTOR('',#6137,1.);
#1784=VECTOR('',#6138,1.);
#1785=VECTOR('',#6139,1.);
#1786=VECTOR('',#6140,1.);
#1787=VECTOR('',#6141,1.);
#1788=VECTOR('',#6142,1.);
#1789=VECTOR('',#6143,1.);
#1790=VECTOR('',#6144,1.);
#1791=VECTOR('',#6145,1.);
#1792=VECTOR('',#6146,1.);
#1793=VECTOR('',#6147,1.);
#1794=VECTOR('',#6148,1.);
#1795=VECTOR('',#6149,1.);
#1796=VECTOR('',#6150,1.);
#1797=VECTOR('',#6151,1.);
#1798=VECTOR('',#6152,1.);
#1799=VECTOR('',#6157,1.);
#1800=VECTOR('',#6158,1.);
#1801=VECTOR('',#6161,1.);
#1802=VECTOR('',#6164,1.);
#1803=VECTOR('',#6167,1.);
#1804=VECTOR('',#6170,1.);
#1805=VECTOR('',#6173,1.);
#1806=VECTOR('',#6174,1.);
#1807=VECTOR('',#6175,1.);
#1808=VECTOR('',#6176,1.);
#1809=VECTOR('',#6179,1.);
#1810=VECTOR('',#6180,1.);
#1811=VECTOR('',#6181,1.);
#1812=VECTOR('',#6182,1.);
#1813=VECTOR('',#6185,1.);
#1814=VECTOR('',#6186,1.);
#1815=VECTOR('',#6187,1.);
#1816=VECTOR('',#6188,1.);
#1817=VECTOR('',#6193,1.);
#1818=VECTOR('',#6194,1.);
#1819=VECTOR('',#6197,1.);
#1820=VECTOR('',#6200,1.);
#1821=VECTOR('',#6203,1.);
#1822=VECTOR('',#6204,1.);
#1823=VECTOR('',#6205,1.);
#1824=VECTOR('',#6206,1.);
#1825=VECTOR('',#6209,1.);
#1826=VECTOR('',#6210,1.);
#1827=VECTOR('',#6213,1.);
#1828=VECTOR('',#6214,1.);
#1829=VECTOR('',#6215,1.);
#1830=VECTOR('',#6218,1.);
#1831=VECTOR('',#6219,1.);
#1832=VECTOR('',#6222,1.);
#1833=VECTOR('',#6223,1.);
#1834=VECTOR('',#6224,1.);
#1835=VECTOR('',#6225,1.);
#1836=VECTOR('',#6226,1.);
#1837=VECTOR('',#6227,1.);
#1838=VECTOR('',#6228,1.);
#1839=VECTOR('',#6229,1.);
#1840=VECTOR('',#6230,1.);
#1841=VECTOR('',#6231,1.);
#1842=VECTOR('',#6232,1.);
#1843=VECTOR('',#6233,1.);
#1844=VECTOR('',#6234,1.);
#1845=VECTOR('',#6235,1.);
#1846=VECTOR('',#6236,1.);
#1847=VECTOR('',#6237,1.);
#1848=VECTOR('',#6240,1.);
#1849=VECTOR('',#6241,1.);
#1850=VECTOR('',#6242,1.);
#1851=VECTOR('',#6245,1.);
#1852=VECTOR('',#6246,1.);
#1853=VECTOR('',#6247,1.);
#1854=VECTOR('',#6248,1.);
#1855=VECTOR('',#6253,1.);
#1856=VECTOR('',#6254,1.);
#1857=VECTOR('',#6255,1.);
#1858=VECTOR('',#6256,1.);
#1859=VECTOR('',#6259,1.);
#1860=VECTOR('',#6260,1.);
#1861=VECTOR('',#6263,1.);
#1862=VECTOR('',#6266,1.);
#1863=VECTOR('',#6279,1.);
#1864=VECTOR('',#6284,1.);
#1865=VECTOR('',#6285,1.);
#1866=VECTOR('',#6302,1.);
#1867=VECTOR('',#6305,1.);
#1868=VECTOR('',#6310,0.0125);
#1869=VECTOR('',#6313,0.00123);
#1870=VECTOR('',#6316,0.00123);
#1871=VECTOR('',#6319,0.00123);
#1872=VECTOR('',#6322,0.00123);
#1873=VECTOR('',#6325,1.);
#1874=VECTOR('',#6326,1.);
#1875=VECTOR('',#6331,1.);
#1876=VECTOR('',#6352,1.);
#1877=VECTOR('',#6353,1.);
#1878=VECTOR('',#6356,1.);
#1879=VECTOR('',#6357,1.);
#1880=VECTOR('',#6358,1.);
#1881=VECTOR('',#6363,1.);
#1882=VECTOR('',#6382,1.);
#1883=VECTOR('',#6383,1.);
#1884=VECTOR('',#6384,1.);
#1885=VECTOR('',#6385,1.);
#1886=VECTOR('',#6386,1.);
#1887=VECTOR('',#6391,1.);
#1888=VECTOR('',#6394,1.);
#1889=VECTOR('',#6397,1.);
#1890=VECTOR('',#6400,1.);
#1891=VECTOR('',#6401,1.);
#1892=VECTOR('',#6404,1.);
#1893=VECTOR('',#6407,1.);
#1894=VECTOR('',#6410,1.);
#1895=VECTOR('',#6413,1.);
#1896=VECTOR('',#6416,1.);
#1897=VECTOR('',#6419,1.);
#1898=VECTOR('',#6422,1.);
#1899=VECTOR('',#6427,1.);
#1900=VECTOR('',#6430,1.);
#1901=VECTOR('',#6431,1.);
#1902=VECTOR('',#6434,1.);
#1903=VECTOR('',#6443,1.);
#1904=VECTOR('',#6446,1.);
#1905=VECTOR('',#6455,1.);
#1906=VECTOR('',#6456,1.);
#1907=VECTOR('',#6475,1.);
#1908=VECTOR('',#6478,1.);
#1909=VECTOR('',#6491,1.);
#1910=VECTOR('',#6494,1.);
#1911=VECTOR('',#6507,1.);
#1912=VECTOR('',#6510,1.);
#1913=VECTOR('',#6523,1.);
#1914=VECTOR('',#6526,1.);
#1915=VECTOR('',#6535,1.);
#1916=VECTOR('',#6536,1.);
#1917=VECTOR('',#6551,1.);
#1918=VECTOR('',#6552,1.);
#1919=VECTOR('',#6567,1.);
#1920=VECTOR('',#6572,1.);
#1921=VECTOR('',#6577,1.);
#1922=VECTOR('',#6582,1.);
#1923=VECTOR('',#6587,1.);
#1924=VECTOR('',#6592,1.);
#1925=VECTOR('',#6597,1.);
#1926=VECTOR('',#6602,1.);
#1927=VECTOR('',#6609,1.);
#1928=VECTOR('',#6610,1.);
#1929=VECTOR('',#6613,1.);
#1930=VECTOR('',#6614,1.);
#1931=VECTOR('',#6615,1.);
#1932=VECTOR('',#6620,1.);
#1933=VECTOR('',#6623,1.);
#1934=VECTOR('',#6624,1.);
#1935=VECTOR('',#6625,1.);
#1936=VECTOR('',#6630,1.);
#1937=VECTOR('',#6639,1.);
#1938=VECTOR('',#6640,1.);
#1939=VECTOR('',#6643,1.);
#1940=VECTOR('',#6644,1.);
#1941=VECTOR('',#6649,1.);
#1942=VECTOR('',#6650,1.);
#1943=VECTOR('',#6653,1.);
#1944=VECTOR('',#6654,1.);
#1945=VECTOR('',#6655,1.);
#1946=VECTOR('',#6660,1.);
#1947=VECTOR('',#6663,1.);
#1948=VECTOR('',#6666,1.);
#1949=VECTOR('',#6669,1.);
#1950=VECTOR('',#6672,1.);
#1951=VECTOR('',#6673,1.);
#1952=VECTOR('',#6674,1.);
#1953=VECTOR('',#6675,1.);
#1954=VECTOR('',#6676,1.);
#1955=VECTOR('',#6681,1.);
#1956=VECTOR('',#6684,1.);
#1957=VECTOR('',#6685,1.);
#1958=VECTOR('',#6688,1.);
#1959=VECTOR('',#6691,1.);
#1960=VECTOR('',#6694,1.);
#1961=VECTOR('',#6697,1.);
#1962=VECTOR('',#6700,1.);
#1963=VECTOR('',#6703,1.);
#1964=VECTOR('',#6706,1.);
#1965=VECTOR('',#6711,1.);
#1966=VECTOR('',#6714,1.);
#1967=VECTOR('',#6715,1.);
#1968=VECTOR('',#6718,1.);
#1969=VECTOR('',#6723,1.);
#1970=VECTOR('',#6726,1.);
#1971=VECTOR('',#6729,1.);
#1972=VECTOR('',#6730,1.);
#1973=VECTOR('',#6735,1.);
#1974=VECTOR('',#6740,1.);
#1975=VECTOR('',#6741,1.);
#1976=VECTOR('',#6742,1.);
#1977=VECTOR('',#6751,1.);
#1978=VECTOR('',#6752,1.);
#1979=VECTOR('',#6753,1.);
#1980=VECTOR('',#6754,1.);
#1981=VECTOR('',#6759,1.);
#1982=VECTOR('',#6764,1.);
#1983=VECTOR('',#6773,1.);
#1984=VECTOR('',#6774,1.);
#1985=VECTOR('',#6779,1.);
#1986=VECTOR('',#6784,1.);
#1987=VECTOR('',#6785,1.);
#1988=VECTOR('',#6786,1.);
#1989=VECTOR('',#6795,1.);
#1990=VECTOR('',#6796,1.);
#1991=VECTOR('',#6797,1.);
#1992=VECTOR('',#6798,1.);
#1993=VECTOR('',#6803,1.);
#1994=VECTOR('',#6808,1.);
#1995=VECTOR('',#6817,1.);
#1996=VECTOR('',#6818,1.);
#1997=VECTOR('',#6819,1.);
#1998=VECTOR('',#6820,1.);
#1999=VECTOR('',#6825,1.);
#2000=VECTOR('',#6830,1.);
#2001=VECTOR('',#6839,1.);
#2002=VECTOR('',#6840,1.);
#2003=VECTOR('',#6841,1.);
#2004=VECTOR('',#6842,1.);
#2005=VECTOR('',#6847,1.);
#2006=VECTOR('',#6852,1.);
#2007=VECTOR('',#6861,1.);
#2008=VECTOR('',#6862,1.);
#2009=VECTOR('',#6863,1.);
#2010=VECTOR('',#6864,1.);
#2011=VECTOR('',#6869,1.);
#2012=VECTOR('',#6874,1.);
#2013=VECTOR('',#6883,1.);
#2014=VECTOR('',#6884,1.);
#2015=VECTOR('',#6889,1.);
#2016=VECTOR('',#6894,1.);
#2017=VECTOR('',#6895,1.);
#2018=VECTOR('',#6896,1.);
#2122=VERTEX_POINT('',#7533);
#2123=VERTEX_POINT('',#7534);
#2124=VERTEX_POINT('',#7536);
#2125=VERTEX_POINT('',#7538);
#2126=VERTEX_POINT('',#7542);
#2127=VERTEX_POINT('',#7543);
#2128=VERTEX_POINT('',#7545);
#2129=VERTEX_POINT('',#7547);
#2130=VERTEX_POINT('',#7554);
#2131=VERTEX_POINT('',#7556);
#2132=VERTEX_POINT('',#7558);
#2133=VERTEX_POINT('',#7560);
#2134=VERTEX_POINT('',#7562);
#2135=VERTEX_POINT('',#7564);
#2136=VERTEX_POINT('',#7568);
#2137=VERTEX_POINT('',#7570);
#2138=VERTEX_POINT('',#7572);
#2139=VERTEX_POINT('',#7574);
#2140=VERTEX_POINT('',#7576);
#2141=VERTEX_POINT('',#7578);
#2142=VERTEX_POINT('',#7582);
#2143=VERTEX_POINT('',#7584);
#2144=VERTEX_POINT('',#7588);
#2145=VERTEX_POINT('',#7589);
#2146=VERTEX_POINT('',#7591);
#2147=VERTEX_POINT('',#7593);
#2148=VERTEX_POINT('',#7597);
#2149=VERTEX_POINT('',#7599);
#2150=VERTEX_POINT('',#7603);
#2151=VERTEX_POINT('',#7604);
#2152=VERTEX_POINT('',#7609);
#2153=VERTEX_POINT('',#7612);
#2154=VERTEX_POINT('',#7613);
#2155=VERTEX_POINT('',#7615);
#2156=VERTEX_POINT('',#7617);
#2157=VERTEX_POINT('',#7620);
#2158=VERTEX_POINT('',#7621);
#2159=VERTEX_POINT('',#7623);
#2160=VERTEX_POINT('',#7625);
#2161=VERTEX_POINT('',#7628);
#2162=VERTEX_POINT('',#7629);
#2163=VERTEX_POINT('',#7631);
#2164=VERTEX_POINT('',#7633);
#2165=VERTEX_POINT('',#7636);
#2166=VERTEX_POINT('',#7637);
#2167=VERTEX_POINT('',#7639);
#2168=VERTEX_POINT('',#7641);
#2169=VERTEX_POINT('',#7644);
#2170=VERTEX_POINT('',#7645);
#2171=VERTEX_POINT('',#7647);
#2172=VERTEX_POINT('',#7649);
#2173=VERTEX_POINT('',#7652);
#2174=VERTEX_POINT('',#7653);
#2175=VERTEX_POINT('',#7655);
#2176=VERTEX_POINT('',#7657);
#2177=VERTEX_POINT('',#7660);
#2178=VERTEX_POINT('',#7661);
#2179=VERTEX_POINT('',#7663);
#2180=VERTEX_POINT('',#7665);
#2181=VERTEX_POINT('',#7668);
#2182=VERTEX_POINT('',#7669);
#2183=VERTEX_POINT('',#7671);
#2184=VERTEX_POINT('',#7673);
#2185=VERTEX_POINT('',#7677);
#2186=VERTEX_POINT('',#7678);
#2187=VERTEX_POINT('',#7680);
#2188=VERTEX_POINT('',#7684);
#2189=VERTEX_POINT('',#7685);
#2190=VERTEX_POINT('',#7687);
#2191=VERTEX_POINT('',#7691);
#2192=VERTEX_POINT('',#7692);
#2193=VERTEX_POINT('',#7694);
#2194=VERTEX_POINT('',#7698);
#2195=VERTEX_POINT('',#7699);
#2196=VERTEX_POINT('',#7701);
#2197=VERTEX_POINT('',#7705);
#2198=VERTEX_POINT('',#7706);
#2199=VERTEX_POINT('',#7708);
#2200=VERTEX_POINT('',#7712);
#2201=VERTEX_POINT('',#7713);
#2202=VERTEX_POINT('',#7715);
#2203=VERTEX_POINT('',#7719);
#2204=VERTEX_POINT('',#7721);
#2205=VERTEX_POINT('',#7725);
#2206=VERTEX_POINT('',#7726);
#2207=VERTEX_POINT('',#7728);
#2208=VERTEX_POINT('',#7732);
#2209=VERTEX_POINT('',#7733);
#2210=VERTEX_POINT('',#7735);
#2211=VERTEX_POINT('',#7739);
#2212=VERTEX_POINT('',#7740);
#2213=VERTEX_POINT('',#7742);
#2214=VERTEX_POINT('',#7746);
#2215=VERTEX_POINT('',#7747);
#2216=VERTEX_POINT('',#7754);
#2217=VERTEX_POINT('',#7758);
#2218=VERTEX_POINT('',#7760);
#2219=VERTEX_POINT('',#7767);
#2220=VERTEX_POINT('',#7770);
#2221=VERTEX_POINT('',#7771);
#2222=VERTEX_POINT('',#7773);
#2223=VERTEX_POINT('',#7775);
#2224=VERTEX_POINT('',#7778);
#2225=VERTEX_POINT('',#7779);
#2226=VERTEX_POINT('',#7781);
#2227=VERTEX_POINT('',#7783);
#2228=VERTEX_POINT('',#7786);
#2229=VERTEX_POINT('',#7787);
#2230=VERTEX_POINT('',#7789);
#2231=VERTEX_POINT('',#7791);
#2232=VERTEX_POINT('',#7794);
#2233=VERTEX_POINT('',#7795);
#2234=VERTEX_POINT('',#7797);
#2235=VERTEX_POINT('',#7799);
#2236=VERTEX_POINT('',#7802);
#2237=VERTEX_POINT('',#7803);
#2238=VERTEX_POINT('',#7805);
#2239=VERTEX_POINT('',#7807);
#2240=VERTEX_POINT('',#7810);
#2241=VERTEX_POINT('',#7811);
#2242=VERTEX_POINT('',#7813);
#2243=VERTEX_POINT('',#7815);
#2244=VERTEX_POINT('',#7818);
#2245=VERTEX_POINT('',#7819);
#2246=VERTEX_POINT('',#7821);
#2247=VERTEX_POINT('',#7823);
#2248=VERTEX_POINT('',#7826);
#2249=VERTEX_POINT('',#7827);
#2250=VERTEX_POINT('',#7829);
#2251=VERTEX_POINT('',#7831);
#2252=VERTEX_POINT('',#7835);
#2253=VERTEX_POINT('',#7836);
#2254=VERTEX_POINT('',#7838);
#2255=VERTEX_POINT('',#7842);
#2256=VERTEX_POINT('',#7843);
#2257=VERTEX_POINT('',#7845);
#2258=VERTEX_POINT('',#7849);
#2259=VERTEX_POINT('',#7850);
#2260=VERTEX_POINT('',#7852);
#2261=VERTEX_POINT('',#7856);
#2262=VERTEX_POINT('',#7857);
#2263=VERTEX_POINT('',#7859);
#2264=VERTEX_POINT('',#7861);
#2265=VERTEX_POINT('',#7865);
#2266=VERTEX_POINT('',#7866);
#2267=VERTEX_POINT('',#7868);
#2268=VERTEX_POINT('',#7870);
#2269=VERTEX_POINT('',#7874);
#2270=VERTEX_POINT('',#7875);
#2271=VERTEX_POINT('',#7877);
#2272=VERTEX_POINT('',#7879);
#2273=VERTEX_POINT('',#7883);
#2274=VERTEX_POINT('',#7884);
#2275=VERTEX_POINT('',#7886);
#2276=VERTEX_POINT('',#7890);
#2277=VERTEX_POINT('',#7891);
#2278=VERTEX_POINT('',#7893);
#2279=VERTEX_POINT('',#7897);
#2280=VERTEX_POINT('',#7898);
#2281=VERTEX_POINT('',#7900);
#2282=VERTEX_POINT('',#7902);
#2283=VERTEX_POINT('',#7909);
#2284=VERTEX_POINT('',#7911);
#2285=VERTEX_POINT('',#7918);
#2286=VERTEX_POINT('',#7919);
#2287=VERTEX_POINT('',#7921);
#2288=VERTEX_POINT('',#7924);
#2289=VERTEX_POINT('',#7926);
#2290=VERTEX_POINT('',#7929);
#2291=VERTEX_POINT('',#7931);
#2292=VERTEX_POINT('',#7934);
#2293=VERTEX_POINT('',#7936);
#2294=VERTEX_POINT('',#7939);
#2295=VERTEX_POINT('',#7941);
#2296=VERTEX_POINT('',#7943);
#2297=VERTEX_POINT('',#7947);
#2298=VERTEX_POINT('',#7949);
#2299=VERTEX_POINT('',#7953);
#2300=VERTEX_POINT('',#7954);
#2301=VERTEX_POINT('',#7960);
#2302=VERTEX_POINT('',#7963);
#2303=VERTEX_POINT('',#7965);
#2304=VERTEX_POINT('',#7968);
#2305=VERTEX_POINT('',#7970);
#2306=VERTEX_POINT('',#7972);
#2307=VERTEX_POINT('',#7978);
#2308=VERTEX_POINT('',#7980);
#2309=VERTEX_POINT('',#7982);
#2310=VERTEX_POINT('',#7984);
#2311=VERTEX_POINT('',#7986);
#2312=VERTEX_POINT('',#7989);
#2313=VERTEX_POINT('',#7992);
#2314=VERTEX_POINT('',#7994);
#2315=VERTEX_POINT('',#7996);
#2316=VERTEX_POINT('',#8000);
#2317=VERTEX_POINT('',#8002);
#2318=VERTEX_POINT('',#8004);
#2319=VERTEX_POINT('',#8006);
#2320=VERTEX_POINT('',#8008);
#2321=VERTEX_POINT('',#8029);
#2322=VERTEX_POINT('',#8041);
#2323=VERTEX_POINT('',#8042);
#2324=VERTEX_POINT('',#8044);
#2325=VERTEX_POINT('',#8048);
#2326=VERTEX_POINT('',#8050);
#2327=VERTEX_POINT('',#8054);
#2328=VERTEX_POINT('',#8072);
#2329=VERTEX_POINT('',#8073);
#2330=VERTEX_POINT('',#8075);
#2331=VERTEX_POINT('',#8077);
#2332=VERTEX_POINT('',#8080);
#2333=VERTEX_POINT('',#8081);
#2334=VERTEX_POINT('',#8083);
#2335=VERTEX_POINT('',#8085);
#2336=VERTEX_POINT('',#8088);
#2337=VERTEX_POINT('',#8089);
#2338=VERTEX_POINT('',#8091);
#2339=VERTEX_POINT('',#8093);
#2340=VERTEX_POINT('',#8096);
#2341=VERTEX_POINT('',#8097);
#2342=VERTEX_POINT('',#8099);
#2343=VERTEX_POINT('',#8101);
#2344=VERTEX_POINT('',#8104);
#2345=VERTEX_POINT('',#8105);
#2346=VERTEX_POINT('',#8107);
#2347=VERTEX_POINT('',#8109);
#2348=VERTEX_POINT('',#8112);
#2349=VERTEX_POINT('',#8113);
#2350=VERTEX_POINT('',#8115);
#2351=VERTEX_POINT('',#8117);
#2352=VERTEX_POINT('',#8120);
#2353=VERTEX_POINT('',#8121);
#2354=VERTEX_POINT('',#8123);
#2355=VERTEX_POINT('',#8125);
#2356=VERTEX_POINT('',#8128);
#2357=VERTEX_POINT('',#8129);
#2358=VERTEX_POINT('',#8131);
#2359=VERTEX_POINT('',#8133);
#2360=VERTEX_POINT('',#8137);
#2361=VERTEX_POINT('',#8144);
#2362=VERTEX_POINT('',#8151);
#2363=VERTEX_POINT('',#8155);
#2364=VERTEX_POINT('',#8159);
#2365=VERTEX_POINT('',#8166);
#2366=VERTEX_POINT('',#8170);
#2367=VERTEX_POINT('',#8177);
#2368=VERTEX_POINT('',#8181);
#2369=VERTEX_POINT('',#8188);
#2370=VERTEX_POINT('',#8192);
#2371=VERTEX_POINT('',#8199);
#2372=VERTEX_POINT('',#8206);
#2373=VERTEX_POINT('',#8210);
#2374=VERTEX_POINT('',#8217);
#2375=VERTEX_POINT('',#8221);
#2376=VERTEX_POINT('',#8249);
#2377=VERTEX_POINT('',#8250);
#2378=VERTEX_POINT('',#8252);
#2379=VERTEX_POINT('',#8256);
#2380=VERTEX_POINT('',#8258);
#2381=VERTEX_POINT('',#8262);
#2382=VERTEX_POINT('',#8266);
#2383=VERTEX_POINT('',#8268);
#2384=VERTEX_POINT('',#8272);
#2385=VERTEX_POINT('',#8278);
#2386=VERTEX_POINT('',#8279);
#2387=VERTEX_POINT('',#8281);
#2388=VERTEX_POINT('',#8288);
#2389=VERTEX_POINT('',#8289);
#2390=VERTEX_POINT('',#8291);
#2391=VERTEX_POINT('',#8295);
#2392=VERTEX_POINT('',#8297);
#2393=VERTEX_POINT('',#8301);
#2394=VERTEX_POINT('',#8317);
#2395=VERTEX_POINT('',#8318);
#2396=VERTEX_POINT('',#8320);
#2397=VERTEX_POINT('',#8322);
#2398=VERTEX_POINT('',#8325);
#2399=VERTEX_POINT('',#8326);
#2400=VERTEX_POINT('',#8328);
#2401=VERTEX_POINT('',#8330);
#2402=VERTEX_POINT('',#8333);
#2403=VERTEX_POINT('',#8334);
#2404=VERTEX_POINT('',#8336);
#2405=VERTEX_POINT('',#8338);
#2406=VERTEX_POINT('',#8341);
#2407=VERTEX_POINT('',#8342);
#2408=VERTEX_POINT('',#8344);
#2409=VERTEX_POINT('',#8346);
#2410=VERTEX_POINT('',#8349);
#2411=VERTEX_POINT('',#8350);
#2412=VERTEX_POINT('',#8352);
#2413=VERTEX_POINT('',#8354);
#2414=VERTEX_POINT('',#8357);
#2415=VERTEX_POINT('',#8358);
#2416=VERTEX_POINT('',#8360);
#2417=VERTEX_POINT('',#8362);
#2418=VERTEX_POINT('',#8365);
#2419=VERTEX_POINT('',#8366);
#2420=VERTEX_POINT('',#8368);
#2421=VERTEX_POINT('',#8370);
#2422=VERTEX_POINT('',#8373);
#2423=VERTEX_POINT('',#8374);
#2424=VERTEX_POINT('',#8376);
#2425=VERTEX_POINT('',#8378);
#2426=VERTEX_POINT('',#8385);
#2427=VERTEX_POINT('',#8387);
#2428=VERTEX_POINT('',#8391);
#2429=VERTEX_POINT('',#8392);
#2430=VERTEX_POINT('',#8400);
#2431=VERTEX_POINT('',#8401);
#2432=VERTEX_POINT('',#8403);
#2433=VERTEX_POINT('',#8405);
#2434=VERTEX_POINT('',#8421);
#2435=VERTEX_POINT('',#8423);
#2436=VERTEX_POINT('',#8427);
#2437=VERTEX_POINT('',#8428);
#2438=VERTEX_POINT('',#8436);
#2439=VERTEX_POINT('',#8437);
#2440=VERTEX_POINT('',#8439);
#2441=VERTEX_POINT('',#8441);
#2442=VERTEX_POINT('',#8454);
#2443=VERTEX_POINT('',#8455);
#2444=VERTEX_POINT('',#8457);
#2445=VERTEX_POINT('',#8459);
#2446=VERTEX_POINT('',#8472);
#2447=VERTEX_POINT('',#8473);
#2448=VERTEX_POINT('',#8475);
#2449=VERTEX_POINT('',#8477);
#2450=VERTEX_POINT('',#8490);
#2451=VERTEX_POINT('',#8491);
#2452=VERTEX_POINT('',#8493);
#2453=VERTEX_POINT('',#8495);
#2454=VERTEX_POINT('',#8511);
#2455=VERTEX_POINT('',#8513);
#2456=VERTEX_POINT('',#8517);
#2457=VERTEX_POINT('',#8518);
#2618=EDGE_CURVE('',#2122,#2123,#1204,.T.);
#2619=EDGE_CURVE('',#2124,#2122,#1205,.T.);
#2620=EDGE_CURVE('',#2125,#2124,#1206,.T.);
#2621=EDGE_CURVE('',#2123,#2125,#1207,.T.);
#2622=EDGE_CURVE('',#2126,#2127,#1208,.T.);
#2623=EDGE_CURVE('',#2128,#2126,#1209,.T.);
#2624=EDGE_CURVE('',#2129,#2128,#1210,.T.);
#2625=EDGE_CURVE('',#2129,#2127,#1211,.T.);
#2626=EDGE_CURVE('',#2127,#2122,#1212,.T.);
#2627=EDGE_CURVE('',#2124,#2129,#1213,.T.);
#2628=EDGE_CURVE('',#2125,#2130,#1214,.T.);
#2629=EDGE_CURVE('',#2131,#2130,#1215,.T.);
#2630=EDGE_CURVE('',#2132,#2131,#1216,.T.);
#2631=EDGE_CURVE('',#2133,#2132,#1217,.T.);
#2632=EDGE_CURVE('',#2133,#2134,#1218,.T.);
#2633=EDGE_CURVE('',#2134,#2135,#1219,.T.);
#2634=EDGE_CURVE('',#2123,#2135,#1220,.T.);
#2635=EDGE_CURVE('',#2136,#2126,#1221,.T.);
#2636=EDGE_CURVE('',#2137,#2136,#1222,.T.);
#2637=EDGE_CURVE('',#2137,#2138,#1223,.T.);
#2638=EDGE_CURVE('',#2138,#2139,#1224,.T.);
#2639=EDGE_CURVE('',#2140,#2139,#1225,.T.);
#2640=EDGE_CURVE('',#2140,#2141,#1226,.T.);
#2641=EDGE_CURVE('',#2141,#2128,#1227,.T.);
#2642=EDGE_CURVE('',#2142,#2135,#1228,.T.);
#2643=EDGE_CURVE('',#2143,#2142,#1229,.T.);
#2644=EDGE_CURVE('',#2143,#2136,#1230,.T.);
#2645=EDGE_CURVE('',#2144,#2145,#1231,.T.);
#2646=EDGE_CURVE('',#2146,#2145,#1232,.T.);
#2647=EDGE_CURVE('',#2147,#2146,#1233,.T.);
#2648=EDGE_CURVE('',#2144,#2147,#1234,.T.);
#2649=EDGE_CURVE('',#2148,#2145,#1235,.T.);
#2650=EDGE_CURVE('',#2149,#2148,#1236,.T.);
#2651=EDGE_CURVE('',#2149,#2146,#1237,.T.);
#2652=EDGE_CURVE('',#2150,#2151,#1238,.T.);
#2653=EDGE_CURVE('',#2151,#2149,#1239,.T.);
#2654=EDGE_CURVE('',#2148,#2150,#1240,.T.);
#2655=EDGE_CURVE('',#2137,#2152,#1241,.T.);
#2656=EDGE_CURVE('',#2152,#2143,#1242,.T.);
#2657=EDGE_CURVE('',#2153,#2154,#1243,.T.);
#2658=EDGE_CURVE('',#2153,#2155,#1244,.F.);
#2659=EDGE_CURVE('',#2155,#2156,#1245,.T.);
#2660=EDGE_CURVE('',#2156,#2154,#1246,.T.);
#2661=EDGE_CURVE('',#2157,#2158,#1247,.T.);
#2662=EDGE_CURVE('',#2157,#2159,#1248,.F.);
#2663=EDGE_CURVE('',#2159,#2160,#1249,.T.);
#2664=EDGE_CURVE('',#2160,#2158,#1250,.T.);
#2665=EDGE_CURVE('',#2161,#2162,#1251,.T.);
#2666=EDGE_CURVE('',#2163,#2162,#1252,.T.);
#2667=EDGE_CURVE('',#2164,#2163,#1253,.T.);
#2668=EDGE_CURVE('',#2164,#2161,#1254,.T.);
#2669=EDGE_CURVE('',#2165,#2166,#1255,.T.);
#2670=EDGE_CURVE('',#2167,#2166,#1256,.T.);
#2671=EDGE_CURVE('',#2168,#2167,#1257,.T.);
#2672=EDGE_CURVE('',#2168,#2165,#1258,.T.);
#2673=EDGE_CURVE('',#2169,#2170,#1259,.T.);
#2674=EDGE_CURVE('',#2171,#2170,#1260,.T.);
#2675=EDGE_CURVE('',#2172,#2171,#1261,.T.);
#2676=EDGE_CURVE('',#2172,#2169,#1262,.T.);
#2677=EDGE_CURVE('',#2173,#2174,#1263,.T.);
#2678=EDGE_CURVE('',#2173,#2175,#1264,.F.);
#2679=EDGE_CURVE('',#2175,#2176,#1265,.T.);
#2680=EDGE_CURVE('',#2176,#2174,#1266,.T.);
#2681=EDGE_CURVE('',#2177,#2178,#1267,.T.);
#2682=EDGE_CURVE('',#2179,#2178,#1268,.T.);
#2683=EDGE_CURVE('',#2180,#2179,#1269,.T.);
#2684=EDGE_CURVE('',#2180,#2177,#1270,.T.);
#2685=EDGE_CURVE('',#2181,#2182,#1271,.T.);
#2686=EDGE_CURVE('',#2183,#2182,#1272,.T.);
#2687=EDGE_CURVE('',#2184,#2183,#1273,.T.);
#2688=EDGE_CURVE('',#2184,#2181,#1274,.T.);
#2689=EDGE_CURVE('',#2185,#2186,#941,.T.);
#2690=EDGE_CURVE('',#2185,#2187,#1275,.T.);
#2691=EDGE_CURVE('',#2187,#2186,#1276,.T.);
#2692=EDGE_CURVE('',#2188,#2189,#1277,.T.);
#2693=EDGE_CURVE('',#2188,#2190,#942,.T.);
#2694=EDGE_CURVE('',#2189,#2190,#1278,.T.);
#2695=EDGE_CURVE('',#2191,#2192,#943,.T.);
#2696=EDGE_CURVE('',#2191,#2193,#1279,.T.);
#2697=EDGE_CURVE('',#2193,#2192,#1280,.T.);
#2698=EDGE_CURVE('',#2194,#2195,#1281,.T.);
#2699=EDGE_CURVE('',#2194,#2196,#944,.T.);
#2700=EDGE_CURVE('',#2195,#2196,#1282,.T.);
#2701=EDGE_CURVE('',#2197,#2198,#945,.T.);
#2702=EDGE_CURVE('',#2199,#2197,#1283,.T.);
#2703=EDGE_CURVE('',#2199,#2198,#1284,.T.);
#2704=EDGE_CURVE('',#2200,#2201,#946,.T.);
#2705=EDGE_CURVE('',#2202,#2200,#1285,.T.);
#2706=EDGE_CURVE('',#2202,#2201,#1286,.T.);
#2707=EDGE_CURVE('',#2200,#2203,#1287,.T.);
#2708=EDGE_CURVE('',#2204,#2203,#1288,.T.);
#2709=EDGE_CURVE('',#2202,#2204,#1289,.T.);
#2710=EDGE_CURVE('',#2205,#2206,#1290,.T.);
#2711=EDGE_CURVE('',#2206,#2207,#947,.T.);
#2712=EDGE_CURVE('',#2205,#2207,#1291,.T.);
#2713=EDGE_CURVE('',#2208,#2209,#948,.T.);
#2714=EDGE_CURVE('',#2208,#2210,#1292,.T.);
#2715=EDGE_CURVE('',#2210,#2209,#1293,.T.);
#2716=EDGE_CURVE('',#2211,#2212,#1294,.T.);
#2717=EDGE_CURVE('',#2211,#2213,#949,.T.);
#2718=EDGE_CURVE('',#2212,#2213,#1295,.T.);
#2719=EDGE_CURVE('',#2214,#2215,#1296,.T.);
#2720=EDGE_CURVE('',#2214,#2188,#1297,.T.);
#2721=EDGE_CURVE('',#2187,#2189,#1298,.T.);
#2722=EDGE_CURVE('',#2185,#2194,#1299,.T.);
#2723=EDGE_CURVE('',#2193,#2195,#1300,.T.);
#2724=EDGE_CURVE('',#2191,#2201,#1301,.T.);
#2725=EDGE_CURVE('',#2204,#2216,#1302,.T.);
#2726=EDGE_CURVE('',#2216,#2211,#1303,.T.);
#2727=EDGE_CURVE('',#2210,#2212,#1304,.T.);
#2728=EDGE_CURVE('',#2217,#2208,#1305,.F.);
#2729=EDGE_CURVE('',#2217,#2218,#1306,.T.);
#2730=EDGE_CURVE('',#2218,#2215,#1307,.T.);
#2731=EDGE_CURVE('',#2140,#2144,#1308,.T.);
#2732=EDGE_CURVE('',#2141,#2147,#1309,.T.);
#2733=EDGE_CURVE('',#2134,#2219,#1310,.T.);
#2734=EDGE_CURVE('',#2219,#2142,#1311,.T.);
#2735=EDGE_CURVE('',#2220,#2221,#1312,.T.);
#2736=EDGE_CURVE('',#2220,#2222,#1313,.F.);
#2737=EDGE_CURVE('',#2222,#2223,#1314,.T.);
#2738=EDGE_CURVE('',#2223,#2221,#1315,.T.);
#2739=EDGE_CURVE('',#2224,#2225,#1316,.T.);
#2740=EDGE_CURVE('',#2226,#2225,#1317,.T.);
#2741=EDGE_CURVE('',#2227,#2226,#1318,.T.);
#2742=EDGE_CURVE('',#2227,#2224,#1319,.T.);
#2743=EDGE_CURVE('',#2228,#2229,#1320,.T.);
#2744=EDGE_CURVE('',#2228,#2230,#1321,.F.);
#2745=EDGE_CURVE('',#2230,#2231,#1322,.T.);
#2746=EDGE_CURVE('',#2231,#2229,#1323,.T.);
#2747=EDGE_CURVE('',#2232,#2233,#1324,.T.);
#2748=EDGE_CURVE('',#2234,#2233,#1325,.T.);
#2749=EDGE_CURVE('',#2235,#2234,#1326,.T.);
#2750=EDGE_CURVE('',#2235,#2232,#1327,.T.);
#2751=EDGE_CURVE('',#2236,#2237,#1328,.T.);
#2752=EDGE_CURVE('',#2238,#2237,#1329,.T.);
#2753=EDGE_CURVE('',#2239,#2238,#1330,.T.);
#2754=EDGE_CURVE('',#2239,#2236,#1331,.T.);
#2755=EDGE_CURVE('',#2240,#2241,#1332,.T.);
#2756=EDGE_CURVE('',#2240,#2242,#1333,.F.);
#2757=EDGE_CURVE('',#2242,#2243,#1334,.T.);
#2758=EDGE_CURVE('',#2243,#2241,#1335,.T.);
#2759=EDGE_CURVE('',#2244,#2245,#1336,.T.);
#2760=EDGE_CURVE('',#2244,#2246,#1337,.F.);
#2761=EDGE_CURVE('',#2246,#2247,#1338,.T.);
#2762=EDGE_CURVE('',#2247,#2245,#1339,.T.);
#2763=EDGE_CURVE('',#2248,#2249,#1340,.T.);
#2764=EDGE_CURVE('',#2248,#2250,#1341,.F.);
#2765=EDGE_CURVE('',#2250,#2251,#1342,.T.);
#2766=EDGE_CURVE('',#2251,#2249,#1343,.T.);
#2767=EDGE_CURVE('',#2252,#2253,#950,.T.);
#2768=EDGE_CURVE('',#2252,#2254,#1344,.T.);
#2769=EDGE_CURVE('',#2254,#2253,#1345,.T.);
#2770=EDGE_CURVE('',#2255,#2256,#1346,.T.);
#2771=EDGE_CURVE('',#2255,#2257,#951,.T.);
#2772=EDGE_CURVE('',#2256,#2257,#1347,.T.);
#2773=EDGE_CURVE('',#2258,#2259,#1348,.T.);
#2774=EDGE_CURVE('',#2258,#2260,#952,.T.);
#2775=EDGE_CURVE('',#2259,#2260,#1349,.T.);
#2776=EDGE_CURVE('',#2261,#2262,#1350,.T.);
#2777=EDGE_CURVE('',#2262,#2263,#1351,.T.);
#2778=EDGE_CURVE('',#2264,#2263,#1352,.T.);
#2779=EDGE_CURVE('',#2261,#2264,#1353,.T.);
#2780=EDGE_CURVE('',#2265,#2266,#1354,.T.);
#2781=EDGE_CURVE('',#2266,#2267,#1355,.T.);
#2782=EDGE_CURVE('',#2268,#2267,#1356,.T.);
#2783=EDGE_CURVE('',#2265,#2268,#1357,.T.);
#2784=EDGE_CURVE('',#2269,#2270,#1358,.T.);
#2785=EDGE_CURVE('',#2270,#2271,#1359,.T.);
#2786=EDGE_CURVE('',#2272,#2271,#1360,.T.);
#2787=EDGE_CURVE('',#2269,#2272,#1361,.T.);
#2788=EDGE_CURVE('',#2273,#2274,#953,.T.);
#2789=EDGE_CURVE('',#2273,#2275,#1362,.T.);
#2790=EDGE_CURVE('',#2275,#2274,#1363,.T.);
#2791=EDGE_CURVE('',#2276,#2277,#1364,.T.);
#2792=EDGE_CURVE('',#2276,#2278,#954,.T.);
#2793=EDGE_CURVE('',#2277,#2278,#1365,.T.);
#2794=EDGE_CURVE('',#2279,#2280,#1366,.T.);
#2795=EDGE_CURVE('',#2280,#2281,#1367,.T.);
#2796=EDGE_CURVE('',#2282,#2281,#1368,.T.);
#2797=EDGE_CURVE('',#2279,#2282,#1369,.T.);
#2798=EDGE_CURVE('',#2253,#2257,#1370,.T.);
#2799=EDGE_CURVE('',#2254,#2256,#1371,.T.);
#2800=EDGE_CURVE('',#2283,#2260,#1372,.T.);
#2801=EDGE_CURVE('',#2284,#2283,#1373,.T.);
#2802=EDGE_CURVE('',#2284,#2259,#1374,.T.);
#2803=EDGE_CURVE('',#2274,#2278,#1375,.T.);
#2804=EDGE_CURVE('',#2275,#2277,#1376,.T.);
#2805=EDGE_CURVE('',#2285,#2286,#1377,.T.);
#2806=EDGE_CURVE('',#2285,#2287,#1378,.T.);
#2807=EDGE_CURVE('',#2279,#2287,#1379,.T.);
#2808=EDGE_CURVE('',#2282,#2288,#1380,.T.);
#2809=EDGE_CURVE('',#2288,#2289,#1381,.T.);
#2810=EDGE_CURVE('',#2269,#2289,#1382,.T.);
#2811=EDGE_CURVE('',#2272,#2290,#1383,.T.);
#2812=EDGE_CURVE('',#2290,#2291,#1384,.T.);
#2813=EDGE_CURVE('',#2265,#2291,#1385,.T.);
#2814=EDGE_CURVE('',#2268,#2292,#1386,.T.);
#2815=EDGE_CURVE('',#2292,#2293,#1387,.T.);
#2816=EDGE_CURVE('',#2261,#2293,#1388,.T.);
#2817=EDGE_CURVE('',#2264,#2294,#1389,.T.);
#2818=EDGE_CURVE('',#2295,#2294,#1390,.F.);
#2819=EDGE_CURVE('',#2295,#2296,#1391,.T.);
#2820=EDGE_CURVE('',#2286,#2296,#1392,.T.);
#2821=EDGE_CURVE('',#2130,#2297,#1393,.T.);
#2822=EDGE_CURVE('',#2297,#2298,#1394,.F.);
#2823=EDGE_CURVE('',#2131,#2298,#1395,.T.);
#2824=EDGE_CURVE('',#2299,#2300,#1396,.T.);
#2825=EDGE_CURVE('',#2299,#2138,#1397,.T.);
#2826=EDGE_CURVE('',#2152,#2219,#1398,.T.);
#2827=EDGE_CURVE('',#2300,#2133,#1399,.T.);
#2828=EDGE_CURVE('',#2301,#2217,#955,.T.);
#2829=EDGE_CURVE('',#2150,#2301,#1400,.T.);
#2830=EDGE_CURVE('',#2139,#2302,#1401,.T.);
#2831=EDGE_CURVE('',#2303,#2302,#1402,.T.);
#2832=EDGE_CURVE('',#2132,#2303,#1403,.T.);
#2833=EDGE_CURVE('',#2298,#2304,#956,.T.);
#2834=EDGE_CURVE('',#2305,#2304,#1404,.T.);
#2835=EDGE_CURVE('',#2305,#2306,#1405,.T.);
#2836=EDGE_CURVE('',#2306,#2285,#957,.T.);
#2837=EDGE_CURVE('',#2218,#2286,#1406,.T.);
#2838=EDGE_CURVE('',#2215,#2296,#1407,.T.);
#2839=EDGE_CURVE('',#2307,#2307,#958,.T.);
#2840=EDGE_CURVE('',#2308,#2308,#959,.T.);
#2841=EDGE_CURVE('',#2309,#2309,#960,.T.);
#2842=EDGE_CURVE('',#2310,#2310,#961,.T.);
#2843=EDGE_CURVE('',#2311,#2311,#962,.T.);
#2844=EDGE_CURVE('',#2151,#2312,#1408,.T.);
#2845=EDGE_CURVE('',#2214,#2312,#963,.T.);
#2846=EDGE_CURVE('',#2313,#2295,#964,.T.);
#2847=EDGE_CURVE('',#2314,#2313,#1409,.T.);
#2848=EDGE_CURVE('',#2314,#2315,#1410,.T.);
#2849=EDGE_CURVE('',#2315,#2297,#965,.F.);
#2850=EDGE_CURVE('',#2316,#2316,#966,.T.);
#2851=EDGE_CURVE('',#2317,#2317,#967,.T.);
#2852=EDGE_CURVE('',#2318,#2318,#968,.T.);
#2853=EDGE_CURVE('',#2319,#2319,#969,.T.);
#2854=EDGE_CURVE('',#2320,#2320,#970,.T.);
#2855=EDGE_CURVE('',#2299,#2302,#1411,.T.);
#2856=EDGE_CURVE('',#2300,#2303,#1412,.T.);
#2857=EDGE_CURVE('',#2320,#2311,#1413,.T.);
#2858=EDGE_CURVE('',#2319,#2310,#1414,.T.);
#2859=EDGE_CURVE('',#2318,#2309,#1415,.T.);
#2860=EDGE_CURVE('',#2317,#2308,#1416,.T.);
#2861=EDGE_CURVE('',#2316,#2307,#1417,.T.);
#2862=EDGE_CURVE('',#2304,#2315,#1418,.T.);
#2863=EDGE_CURVE('',#2305,#2314,#1419,.T.);
#2864=EDGE_CURVE('',#2321,#2283,#971,.T.);
#2865=EDGE_CURVE('',#2321,#2284,#1420,.T.);
#2866=EDGE_CURVE('',#2262,#2293,#972,.T.);
#2867=EDGE_CURVE('',#2263,#2294,#973,.T.);
#2868=EDGE_CURVE('',#2266,#2291,#974,.T.);
#2869=EDGE_CURVE('',#2267,#2292,#975,.T.);
#2870=EDGE_CURVE('',#2322,#2323,#976,.T.);
#2871=EDGE_CURVE('',#2324,#2322,#1421,.T.);
#2872=EDGE_CURVE('',#2324,#2323,#1422,.T.);
#2873=EDGE_CURVE('',#2322,#2325,#1423,.F.);
#2874=EDGE_CURVE('',#2326,#2325,#1424,.T.);
#2875=EDGE_CURVE('',#2324,#2326,#1425,.T.);
#2876=EDGE_CURVE('',#2325,#2327,#977,.T.);
#2877=EDGE_CURVE('',#2326,#2327,#1426,.T.);
#2878=EDGE_CURVE('',#2270,#2289,#978,.T.);
#2879=EDGE_CURVE('',#2271,#2290,#979,.T.);
#2880=EDGE_CURVE('',#2280,#2287,#980,.T.);
#2881=EDGE_CURVE('',#2281,#2288,#981,.T.);
#2882=EDGE_CURVE('',#2306,#2273,#1427,.T.);
#2883=EDGE_CURVE('',#2255,#2313,#1428,.T.);
#2884=EDGE_CURVE('',#2258,#2252,#1429,.T.);
#2885=EDGE_CURVE('',#2323,#2321,#1430,.T.);
#2886=EDGE_CURVE('',#2276,#2327,#1431,.T.);
#2887=EDGE_CURVE('',#2328,#2329,#982,.T.);
#2888=EDGE_CURVE('',#2329,#2330,#1432,.T.);
#2889=EDGE_CURVE('',#2331,#2330,#983,.T.);
#2890=EDGE_CURVE('',#2331,#2328,#1433,.F.);
#2891=EDGE_CURVE('',#2332,#2333,#984,.T.);
#2892=EDGE_CURVE('',#2333,#2334,#1434,.T.);
#2893=EDGE_CURVE('',#2335,#2334,#985,.T.);
#2894=EDGE_CURVE('',#2335,#2332,#1435,.F.);
#2895=EDGE_CURVE('',#2336,#2337,#1436,.F.);
#2896=EDGE_CURVE('',#2337,#2338,#986,.T.);
#2897=EDGE_CURVE('',#2339,#2338,#1437,.F.);
#2898=EDGE_CURVE('',#2336,#2339,#987,.T.);
#2899=EDGE_CURVE('',#2340,#2341,#1438,.F.);
#2900=EDGE_CURVE('',#2341,#2342,#988,.T.);
#2901=EDGE_CURVE('',#2343,#2342,#1439,.F.);
#2902=EDGE_CURVE('',#2340,#2343,#989,.T.);
#2903=EDGE_CURVE('',#2344,#2345,#1440,.T.);
#2904=EDGE_CURVE('',#2345,#2346,#990,.T.);
#2905=EDGE_CURVE('',#2347,#2346,#1441,.T.);
#2906=EDGE_CURVE('',#2344,#2347,#991,.T.);
#2907=EDGE_CURVE('',#2348,#2349,#1442,.F.);
#2908=EDGE_CURVE('',#2349,#2350,#992,.T.);
#2909=EDGE_CURVE('',#2351,#2350,#1443,.F.);
#2910=EDGE_CURVE('',#2348,#2351,#993,.T.);
#2911=EDGE_CURVE('',#2352,#2353,#994,.T.);
#2912=EDGE_CURVE('',#2353,#2354,#1444,.T.);
#2913=EDGE_CURVE('',#2355,#2354,#995,.T.);
#2914=EDGE_CURVE('',#2355,#2352,#1445,.F.);
#2915=EDGE_CURVE('',#2356,#2357,#1446,.F.);
#2916=EDGE_CURVE('',#2357,#2358,#996,.T.);
#2917=EDGE_CURVE('',#2359,#2358,#1447,.F.);
#2918=EDGE_CURVE('',#2356,#2359,#997,.T.);
#2919=EDGE_CURVE('',#2222,#2360,#998,.T.);
#2920=EDGE_CURVE('',#2360,#2356,#999,.T.);
#2921=EDGE_CURVE('',#2359,#2223,#1448,.T.);
#2922=EDGE_CURVE('',#2358,#2221,#1449,.T.);
#2923=EDGE_CURVE('',#2357,#2361,#1000,.F.);
#2924=EDGE_CURVE('',#2361,#2220,#1001,.F.);
#2925=EDGE_CURVE('',#2355,#2227,#1450,.T.);
#2926=EDGE_CURVE('',#2352,#2226,#1451,.T.);
#2927=EDGE_CURVE('',#2354,#2362,#1002,.T.);
#2928=EDGE_CURVE('',#2362,#2224,#1003,.T.);
#2929=EDGE_CURVE('',#2225,#2363,#1004,.F.);
#2930=EDGE_CURVE('',#2363,#2353,#1005,.F.);
#2931=EDGE_CURVE('',#2250,#2364,#1006,.T.);
#2932=EDGE_CURVE('',#2364,#2348,#1007,.T.);
#2933=EDGE_CURVE('',#2351,#2251,#1452,.T.);
#2934=EDGE_CURVE('',#2350,#2249,#1453,.T.);
#2935=EDGE_CURVE('',#2349,#2365,#1008,.F.);
#2936=EDGE_CURVE('',#2365,#2248,#1009,.F.);
#2937=EDGE_CURVE('',#2230,#2366,#1010,.T.);
#2938=EDGE_CURVE('',#2366,#2344,#1011,.T.);
#2939=EDGE_CURVE('',#2347,#2231,#1454,.T.);
#2940=EDGE_CURVE('',#2346,#2229,#1455,.T.);
#2941=EDGE_CURVE('',#2345,#2367,#1012,.F.);
#2942=EDGE_CURVE('',#2367,#2228,#1013,.F.);
#2943=EDGE_CURVE('',#2246,#2368,#1014,.T.);
#2944=EDGE_CURVE('',#2368,#2340,#1015,.T.);
#2945=EDGE_CURVE('',#2343,#2247,#1456,.T.);
#2946=EDGE_CURVE('',#2342,#2245,#1457,.T.);
#2947=EDGE_CURVE('',#2341,#2369,#1016,.F.);
#2948=EDGE_CURVE('',#2369,#2244,#1017,.F.);
#2949=EDGE_CURVE('',#2242,#2370,#1018,.T.);
#2950=EDGE_CURVE('',#2370,#2336,#1019,.T.);
#2951=EDGE_CURVE('',#2339,#2243,#1458,.T.);
#2952=EDGE_CURVE('',#2338,#2241,#1459,.T.);
#2953=EDGE_CURVE('',#2337,#2371,#1020,.F.);
#2954=EDGE_CURVE('',#2371,#2240,#1021,.F.);
#2955=EDGE_CURVE('',#2335,#2235,#1460,.T.);
#2956=EDGE_CURVE('',#2332,#2234,#1461,.T.);
#2957=EDGE_CURVE('',#2334,#2372,#1022,.T.);
#2958=EDGE_CURVE('',#2372,#2232,#1023,.T.);
#2959=EDGE_CURVE('',#2233,#2373,#1024,.F.);
#2960=EDGE_CURVE('',#2373,#2333,#1025,.F.);
#2961=EDGE_CURVE('',#2331,#2239,#1462,.T.);
#2962=EDGE_CURVE('',#2328,#2238,#1463,.T.);
#2963=EDGE_CURVE('',#2330,#2374,#1026,.T.);
#2964=EDGE_CURVE('',#2374,#2236,#1027,.T.);
#2965=EDGE_CURVE('',#2237,#2375,#1028,.F.);
#2966=EDGE_CURVE('',#2375,#2329,#1029,.F.);
#2967=EDGE_CURVE('',#2365,#2364,#1464,.T.);
#2968=EDGE_CURVE('',#2369,#2368,#1465,.T.);
#2969=EDGE_CURVE('',#2371,#2370,#1466,.T.);
#2970=EDGE_CURVE('',#2374,#2375,#1467,.F.);
#2971=EDGE_CURVE('',#2372,#2373,#1468,.F.);
#2972=EDGE_CURVE('',#2367,#2366,#1469,.F.);
#2973=EDGE_CURVE('',#2362,#2363,#1470,.F.);
#2974=EDGE_CURVE('',#2361,#2360,#1471,.T.);
#2975=EDGE_CURVE('',#2376,#2377,#1030,.T.);
#2976=EDGE_CURVE('',#2378,#2376,#1472,.T.);
#2977=EDGE_CURVE('',#2378,#2377,#1473,.T.);
#2978=EDGE_CURVE('',#2376,#2379,#1474,.F.);
#2979=EDGE_CURVE('',#2380,#2379,#1475,.T.);
#2980=EDGE_CURVE('',#2378,#2380,#1476,.T.);
#2981=EDGE_CURVE('',#2379,#2381,#1031,.T.);
#2982=EDGE_CURVE('',#2380,#2381,#1477,.T.);
#2983=EDGE_CURVE('',#2197,#2382,#1478,.F.);
#2984=EDGE_CURVE('',#2383,#2382,#1479,.T.);
#2985=EDGE_CURVE('',#2199,#2383,#1480,.T.);
#2986=EDGE_CURVE('',#2382,#2384,#1032,.T.);
#2987=EDGE_CURVE('',#2383,#2384,#1481,.T.);
#2988=EDGE_CURVE('',#2203,#2216,#1033,.T.);
#2989=EDGE_CURVE('',#2385,#2386,#1034,.T.);
#2990=EDGE_CURVE('',#2387,#2385,#1482,.T.);
#2991=EDGE_CURVE('',#2387,#2386,#1483,.T.);
#2992=EDGE_CURVE('',#2385,#2206,#1484,.F.);
#2993=EDGE_CURVE('',#2387,#2205,#1485,.T.);
#2994=EDGE_CURVE('',#2388,#2389,#1035,.T.);
#2995=EDGE_CURVE('',#2390,#2388,#1486,.T.);
#2996=EDGE_CURVE('',#2390,#2389,#1487,.T.);
#2997=EDGE_CURVE('',#2388,#2391,#1488,.F.);
#2998=EDGE_CURVE('',#2392,#2391,#1489,.T.);
#2999=EDGE_CURVE('',#2390,#2392,#1490,.T.);
#3000=EDGE_CURVE('',#2391,#2393,#1036,.T.);
#3001=EDGE_CURVE('',#2392,#2393,#1491,.T.);
#3002=EDGE_CURVE('',#2192,#2196,#1492,.F.);
#3003=EDGE_CURVE('',#2209,#2213,#1493,.F.);
#3004=EDGE_CURVE('',#2186,#2190,#1494,.F.);
#3005=EDGE_CURVE('',#2312,#2381,#1495,.T.);
#3006=EDGE_CURVE('',#2389,#2301,#1496,.T.);
#3007=EDGE_CURVE('',#2386,#2393,#1497,.T.);
#3008=EDGE_CURVE('',#2198,#2207,#1498,.T.);
#3009=EDGE_CURVE('',#2377,#2384,#1499,.T.);
#3010=EDGE_CURVE('',#2394,#2395,#1037,.T.);
#3011=EDGE_CURVE('',#2395,#2396,#1500,.F.);
#3012=EDGE_CURVE('',#2397,#2396,#1038,.T.);
#3013=EDGE_CURVE('',#2397,#2394,#1501,.T.);
#3014=EDGE_CURVE('',#2398,#2399,#1502,.T.);
#3015=EDGE_CURVE('',#2399,#2400,#1039,.T.);
#3016=EDGE_CURVE('',#2401,#2400,#1503,.T.);
#3017=EDGE_CURVE('',#2398,#2401,#1040,.T.);
#3018=EDGE_CURVE('',#2402,#2403,#1504,.T.);
#3019=EDGE_CURVE('',#2403,#2404,#1041,.T.);
#3020=EDGE_CURVE('',#2405,#2404,#1505,.T.);
#3021=EDGE_CURVE('',#2402,#2405,#1042,.T.);
#3022=EDGE_CURVE('',#2406,#2407,#1506,.F.);
#3023=EDGE_CURVE('',#2407,#2408,#1043,.T.);
#3024=EDGE_CURVE('',#2409,#2408,#1507,.F.);
#3025=EDGE_CURVE('',#2406,#2409,#1044,.T.);
#3026=EDGE_CURVE('',#2410,#2411,#1508,.T.);
#3027=EDGE_CURVE('',#2411,#2412,#1045,.T.);
#3028=EDGE_CURVE('',#2413,#2412,#1509,.T.);
#3029=EDGE_CURVE('',#2410,#2413,#1046,.T.);
#3030=EDGE_CURVE('',#2414,#2415,#1047,.T.);
#3031=EDGE_CURVE('',#2415,#2416,#1510,.F.);
#3032=EDGE_CURVE('',#2417,#2416,#1048,.T.);
#3033=EDGE_CURVE('',#2417,#2414,#1511,.T.);
#3034=EDGE_CURVE('',#2418,#2419,#1512,.T.);
#3035=EDGE_CURVE('',#2419,#2420,#1049,.T.);
#3036=EDGE_CURVE('',#2421,#2420,#1513,.T.);
#3037=EDGE_CURVE('',#2418,#2421,#1050,.T.);
#3038=EDGE_CURVE('',#2422,#2423,#1051,.T.);
#3039=EDGE_CURVE('',#2423,#2424,#1514,.F.);
#3040=EDGE_CURVE('',#2425,#2424,#1052,.T.);
#3041=EDGE_CURVE('',#2425,#2422,#1515,.T.);
#3042=EDGE_CURVE('',#2425,#2174,#1516,.T.);
#3043=EDGE_CURVE('',#2422,#2176,#1517,.T.);
#3044=EDGE_CURVE('',#2424,#2426,#1053,.T.);
#3045=EDGE_CURVE('',#2426,#2427,#1518,.T.);
#3046=EDGE_CURVE('',#2427,#2173,#1054,.T.);
#3047=EDGE_CURVE('',#2428,#2429,#1519,.T.);
#3048=EDGE_CURVE('',#2429,#2427,#1520,.T.);
#3049=EDGE_CURVE('',#2426,#2428,#1521,.T.);
#3050=EDGE_CURVE('',#2175,#2429,#1055,.F.);
#3051=EDGE_CURVE('',#2428,#2423,#1056,.F.);
#3052=EDGE_CURVE('',#2430,#2431,#1522,.T.);
#3053=EDGE_CURVE('',#2431,#2432,#1523,.F.);
#3054=EDGE_CURVE('',#2433,#2432,#1524,.T.);
#3055=EDGE_CURVE('',#2433,#2430,#1525,.T.);
#3056=EDGE_CURVE('',#2430,#2418,#1057,.T.);
#3057=EDGE_CURVE('',#2421,#2183,#1526,.T.);
#3058=EDGE_CURVE('',#2182,#2431,#1058,.T.);
#3059=EDGE_CURVE('',#2420,#2184,#1527,.T.);
#3060=EDGE_CURVE('',#2419,#2433,#1059,.F.);
#3061=EDGE_CURVE('',#2432,#2181,#1060,.F.);
#3062=EDGE_CURVE('',#2417,#2154,#1528,.T.);
#3063=EDGE_CURVE('',#2414,#2156,#1529,.T.);
#3064=EDGE_CURVE('',#2416,#2434,#1061,.T.);
#3065=EDGE_CURVE('',#2434,#2435,#1530,.T.);
#3066=EDGE_CURVE('',#2435,#2153,#1062,.T.);
#3067=EDGE_CURVE('',#2436,#2437,#1531,.T.);
#3068=EDGE_CURVE('',#2437,#2435,#1532,.T.);
#3069=EDGE_CURVE('',#2434,#2436,#1533,.T.);
#3070=EDGE_CURVE('',#2155,#2437,#1063,.F.);
#3071=EDGE_CURVE('',#2436,#2415,#1064,.F.);
#3072=EDGE_CURVE('',#2438,#2439,#1534,.T.);
#3073=EDGE_CURVE('',#2439,#2440,#1535,.F.);
#3074=EDGE_CURVE('',#2441,#2440,#1536,.T.);
#3075=EDGE_CURVE('',#2441,#2438,#1537,.T.);
#3076=EDGE_CURVE('',#2438,#2410,#1065,.T.);
#3077=EDGE_CURVE('',#2413,#2167,#1538,.T.);
#3078=EDGE_CURVE('',#2166,#2439,#1066,.T.);
#3079=EDGE_CURVE('',#2412,#2168,#1539,.T.);
#3080=EDGE_CURVE('',#2411,#2441,#1067,.F.);
#3081=EDGE_CURVE('',#2440,#2165,#1068,.F.);
#3082=EDGE_CURVE('',#2442,#2443,#1540,.T.);
#3083=EDGE_CURVE('',#2443,#2444,#1541,.F.);
#3084=EDGE_CURVE('',#2445,#2444,#1542,.T.);
#3085=EDGE_CURVE('',#2445,#2442,#1543,.F.);
#3086=EDGE_CURVE('',#2442,#2406,#1069,.T.);
#3087=EDGE_CURVE('',#2409,#2179,#1544,.T.);
#3088=EDGE_CURVE('',#2178,#2443,#1070,.T.);
#3089=EDGE_CURVE('',#2408,#2180,#1545,.T.);
#3090=EDGE_CURVE('',#2407,#2445,#1071,.F.);
#3091=EDGE_CURVE('',#2444,#2177,#1072,.F.);
#3092=EDGE_CURVE('',#2446,#2447,#1546,.T.);
#3093=EDGE_CURVE('',#2447,#2448,#1547,.F.);
#3094=EDGE_CURVE('',#2449,#2448,#1548,.T.);
#3095=EDGE_CURVE('',#2449,#2446,#1549,.T.);
#3096=EDGE_CURVE('',#2446,#2402,#1073,.T.);
#3097=EDGE_CURVE('',#2405,#2171,#1550,.T.);
#3098=EDGE_CURVE('',#2170,#2447,#1074,.T.);
#3099=EDGE_CURVE('',#2404,#2172,#1551,.T.);
#3100=EDGE_CURVE('',#2403,#2449,#1075,.F.);
#3101=EDGE_CURVE('',#2448,#2169,#1076,.F.);
#3102=EDGE_CURVE('',#2450,#2451,#1552,.T.);
#3103=EDGE_CURVE('',#2451,#2452,#1553,.F.);
#3104=EDGE_CURVE('',#2453,#2452,#1554,.T.);
#3105=EDGE_CURVE('',#2453,#2450,#1555,.T.);
#3106=EDGE_CURVE('',#2450,#2398,#1077,.T.);
#3107=EDGE_CURVE('',#2401,#2163,#1556,.T.);
#3108=EDGE_CURVE('',#2162,#2451,#1078,.T.);
#3109=EDGE_CURVE('',#2400,#2164,#1557,.T.);
#3110=EDGE_CURVE('',#2399,#2453,#1079,.F.);
#3111=EDGE_CURVE('',#2452,#2161,#1080,.F.);
#3112=EDGE_CURVE('',#2397,#2158,#1558,.T.);
#3113=EDGE_CURVE('',#2394,#2160,#1559,.T.);
#3114=EDGE_CURVE('',#2396,#2454,#1081,.T.);
#3115=EDGE_CURVE('',#2454,#2455,#1560,.T.);
#3116=EDGE_CURVE('',#2455,#2157,#1082,.T.);
#3117=EDGE_CURVE('',#2456,#2457,#1561,.T.);
#3118=EDGE_CURVE('',#2457,#2455,#1562,.T.);
#3119=EDGE_CURVE('',#2454,#2456,#1563,.T.);
#3120=EDGE_CURVE('',#2159,#2457,#1083,.F.);
#3121=EDGE_CURVE('',#2456,#2395,#1084,.F.);
#3395=ORIENTED_EDGE('',*,*,#2618,.F.);
#3396=ORIENTED_EDGE('',*,*,#2619,.F.);
#3397=ORIENTED_EDGE('',*,*,#2620,.F.);
#3398=ORIENTED_EDGE('',*,*,#2621,.F.);
#3399=ORIENTED_EDGE('',*,*,#2622,.F.);
#3400=ORIENTED_EDGE('',*,*,#2623,.F.);
#3401=ORIENTED_EDGE('',*,*,#2624,.F.);
#3402=ORIENTED_EDGE('',*,*,#2625,.T.);
#3403=ORIENTED_EDGE('',*,*,#2626,.F.);
#3404=ORIENTED_EDGE('',*,*,#2625,.F.);
#3405=ORIENTED_EDGE('',*,*,#2627,.F.);
#3406=ORIENTED_EDGE('',*,*,#2619,.T.);
#3407=ORIENTED_EDGE('',*,*,#2621,.T.);
#3408=ORIENTED_EDGE('',*,*,#2628,.T.);
#3409=ORIENTED_EDGE('',*,*,#2629,.F.);
#3410=ORIENTED_EDGE('',*,*,#2630,.F.);
#3411=ORIENTED_EDGE('',*,*,#2631,.F.);
#3412=ORIENTED_EDGE('',*,*,#2632,.T.);
#3413=ORIENTED_EDGE('',*,*,#2633,.T.);
#3414=ORIENTED_EDGE('',*,*,#2634,.F.);
#3415=ORIENTED_EDGE('',*,*,#2623,.T.);
#3416=ORIENTED_EDGE('',*,*,#2635,.F.);
#3417=ORIENTED_EDGE('',*,*,#2636,.F.);
#3418=ORIENTED_EDGE('',*,*,#2637,.T.);
#3419=ORIENTED_EDGE('',*,*,#2638,.T.);
#3420=ORIENTED_EDGE('',*,*,#2639,.F.);
#3421=ORIENTED_EDGE('',*,*,#2640,.T.);
#3422=ORIENTED_EDGE('',*,*,#2641,.T.);
#3423=ORIENTED_EDGE('',*,*,#2622,.T.);
#3424=ORIENTED_EDGE('',*,*,#2626,.T.);
#3425=ORIENTED_EDGE('',*,*,#2618,.T.);
#3426=ORIENTED_EDGE('',*,*,#2634,.T.);
#3427=ORIENTED_EDGE('',*,*,#2642,.F.);
#3428=ORIENTED_EDGE('',*,*,#2643,.F.);
#3429=ORIENTED_EDGE('',*,*,#2644,.T.);
#3430=ORIENTED_EDGE('',*,*,#2635,.T.);
#3431=ORIENTED_EDGE('',*,*,#2645,.T.);
#3432=ORIENTED_EDGE('',*,*,#2646,.F.);
#3433=ORIENTED_EDGE('',*,*,#2647,.F.);
#3434=ORIENTED_EDGE('',*,*,#2648,.F.);
#3435=ORIENTED_EDGE('',*,*,#2646,.T.);
#3436=ORIENTED_EDGE('',*,*,#2649,.F.);
#3437=ORIENTED_EDGE('',*,*,#2650,.F.);
#3438=ORIENTED_EDGE('',*,*,#2651,.T.);
#3439=ORIENTED_EDGE('',*,*,#2652,.T.);
#3440=ORIENTED_EDGE('',*,*,#2653,.T.);
#3441=ORIENTED_EDGE('',*,*,#2650,.T.);
#3442=ORIENTED_EDGE('',*,*,#2654,.T.);
#3443=ORIENTED_EDGE('',*,*,#2655,.F.);
#3444=ORIENTED_EDGE('',*,*,#2636,.T.);
#3445=ORIENTED_EDGE('',*,*,#2644,.F.);
#3446=ORIENTED_EDGE('',*,*,#2656,.F.);
#3447=ORIENTED_EDGE('',*,*,#2657,.F.);
#3448=ORIENTED_EDGE('',*,*,#2658,.T.);
#3449=ORIENTED_EDGE('',*,*,#2659,.T.);
#3450=ORIENTED_EDGE('',*,*,#2660,.T.);
#3451=ORIENTED_EDGE('',*,*,#2661,.F.);
#3452=ORIENTED_EDGE('',*,*,#2662,.T.);
#3453=ORIENTED_EDGE('',*,*,#2663,.T.);
#3454=ORIENTED_EDGE('',*,*,#2664,.T.);
#3455=ORIENTED_EDGE('',*,*,#2665,.T.);
#3456=ORIENTED_EDGE('',*,*,#2666,.F.);
#3457=ORIENTED_EDGE('',*,*,#2667,.F.);
#3458=ORIENTED_EDGE('',*,*,#2668,.T.);
#3459=ORIENTED_EDGE('',*,*,#2669,.T.);
#3460=ORIENTED_EDGE('',*,*,#2670,.F.);
#3461=ORIENTED_EDGE('',*,*,#2671,.F.);
#3462=ORIENTED_EDGE('',*,*,#2672,.T.);
#3463=ORIENTED_EDGE('',*,*,#2673,.T.);
#3464=ORIENTED_EDGE('',*,*,#2674,.F.);
#3465=ORIENTED_EDGE('',*,*,#2675,.F.);
#3466=ORIENTED_EDGE('',*,*,#2676,.T.);
#3467=ORIENTED_EDGE('',*,*,#2677,.F.);
#3468=ORIENTED_EDGE('',*,*,#2678,.T.);
#3469=ORIENTED_EDGE('',*,*,#2679,.T.);
#3470=ORIENTED_EDGE('',*,*,#2680,.T.);
#3471=ORIENTED_EDGE('',*,*,#2681,.T.);
#3472=ORIENTED_EDGE('',*,*,#2682,.F.);
#3473=ORIENTED_EDGE('',*,*,#2683,.F.);
#3474=ORIENTED_EDGE('',*,*,#2684,.T.);
#3475=ORIENTED_EDGE('',*,*,#2685,.T.);
#3476=ORIENTED_EDGE('',*,*,#2686,.F.);
#3477=ORIENTED_EDGE('',*,*,#2687,.F.);
#3478=ORIENTED_EDGE('',*,*,#2688,.T.);
#3479=ORIENTED_EDGE('',*,*,#2689,.F.);
#3480=ORIENTED_EDGE('',*,*,#2690,.T.);
#3481=ORIENTED_EDGE('',*,*,#2691,.T.);
#3482=ORIENTED_EDGE('',*,*,#2692,.F.);
#3483=ORIENTED_EDGE('',*,*,#2693,.T.);
#3484=ORIENTED_EDGE('',*,*,#2694,.F.);
#3485=ORIENTED_EDGE('',*,*,#2695,.F.);
#3486=ORIENTED_EDGE('',*,*,#2696,.T.);
#3487=ORIENTED_EDGE('',*,*,#2697,.T.);
#3488=ORIENTED_EDGE('',*,*,#2698,.F.);
#3489=ORIENTED_EDGE('',*,*,#2699,.T.);
#3490=ORIENTED_EDGE('',*,*,#2700,.F.);
#3491=ORIENTED_EDGE('',*,*,#2701,.F.);
#3492=ORIENTED_EDGE('',*,*,#2702,.F.);
#3493=ORIENTED_EDGE('',*,*,#2703,.T.);
#3494=ORIENTED_EDGE('',*,*,#2704,.F.);
#3495=ORIENTED_EDGE('',*,*,#2705,.F.);
#3496=ORIENTED_EDGE('',*,*,#2706,.T.);
#3497=ORIENTED_EDGE('',*,*,#2705,.T.);
#3498=ORIENTED_EDGE('',*,*,#2707,.T.);
#3499=ORIENTED_EDGE('',*,*,#2708,.F.);
#3500=ORIENTED_EDGE('',*,*,#2709,.F.);
#3501=ORIENTED_EDGE('',*,*,#2710,.T.);
#3502=ORIENTED_EDGE('',*,*,#2711,.T.);
#3503=ORIENTED_EDGE('',*,*,#2712,.F.);
#3504=ORIENTED_EDGE('',*,*,#2713,.F.);
#3505=ORIENTED_EDGE('',*,*,#2714,.T.);
#3506=ORIENTED_EDGE('',*,*,#2715,.T.);
#3507=ORIENTED_EDGE('',*,*,#2716,.F.);
#3508=ORIENTED_EDGE('',*,*,#2717,.T.);
#3509=ORIENTED_EDGE('',*,*,#2718,.F.);
#3510=ORIENTED_EDGE('',*,*,#2719,.F.);
#3511=ORIENTED_EDGE('',*,*,#2720,.T.);
#3512=ORIENTED_EDGE('',*,*,#2692,.T.);
#3513=ORIENTED_EDGE('',*,*,#2721,.F.);
#3514=ORIENTED_EDGE('',*,*,#2690,.F.);
#3515=ORIENTED_EDGE('',*,*,#2722,.T.);
#3516=ORIENTED_EDGE('',*,*,#2698,.T.);
#3517=ORIENTED_EDGE('',*,*,#2723,.F.);
#3518=ORIENTED_EDGE('',*,*,#2696,.F.);
#3519=ORIENTED_EDGE('',*,*,#2724,.T.);
#3520=ORIENTED_EDGE('',*,*,#2706,.F.);
#3521=ORIENTED_EDGE('',*,*,#2709,.T.);
#3522=ORIENTED_EDGE('',*,*,#2725,.T.);
#3523=ORIENTED_EDGE('',*,*,#2726,.T.);
#3524=ORIENTED_EDGE('',*,*,#2716,.T.);
#3525=ORIENTED_EDGE('',*,*,#2727,.F.);
#3526=ORIENTED_EDGE('',*,*,#2714,.F.);
#3527=ORIENTED_EDGE('',*,*,#2728,.F.);
#3528=ORIENTED_EDGE('',*,*,#2729,.T.);
#3529=ORIENTED_EDGE('',*,*,#2730,.T.);
#3530=ORIENTED_EDGE('',*,*,#2731,.T.);
#3531=ORIENTED_EDGE('',*,*,#2648,.T.);
#3532=ORIENTED_EDGE('',*,*,#2732,.F.);
#3533=ORIENTED_EDGE('',*,*,#2640,.F.);
#3534=ORIENTED_EDGE('',*,*,#2633,.F.);
#3535=ORIENTED_EDGE('',*,*,#2733,.T.);
#3536=ORIENTED_EDGE('',*,*,#2734,.T.);
#3537=ORIENTED_EDGE('',*,*,#2642,.T.);
#3538=ORIENTED_EDGE('',*,*,#2735,.F.);
#3539=ORIENTED_EDGE('',*,*,#2736,.T.);
#3540=ORIENTED_EDGE('',*,*,#2737,.T.);
#3541=ORIENTED_EDGE('',*,*,#2738,.T.);
#3542=ORIENTED_EDGE('',*,*,#2739,.T.);
#3543=ORIENTED_EDGE('',*,*,#2740,.F.);
#3544=ORIENTED_EDGE('',*,*,#2741,.F.);
#3545=ORIENTED_EDGE('',*,*,#2742,.T.);
#3546=ORIENTED_EDGE('',*,*,#2743,.F.);
#3547=ORIENTED_EDGE('',*,*,#2744,.T.);
#3548=ORIENTED_EDGE('',*,*,#2745,.T.);
#3549=ORIENTED_EDGE('',*,*,#2746,.T.);
#3550=ORIENTED_EDGE('',*,*,#2747,.T.);
#3551=ORIENTED_EDGE('',*,*,#2748,.F.);
#3552=ORIENTED_EDGE('',*,*,#2749,.F.);
#3553=ORIENTED_EDGE('',*,*,#2750,.T.);
#3554=ORIENTED_EDGE('',*,*,#2751,.T.);
#3555=ORIENTED_EDGE('',*,*,#2752,.F.);
#3556=ORIENTED_EDGE('',*,*,#2753,.F.);
#3557=ORIENTED_EDGE('',*,*,#2754,.T.);
#3558=ORIENTED_EDGE('',*,*,#2755,.F.);
#3559=ORIENTED_EDGE('',*,*,#2756,.T.);
#3560=ORIENTED_EDGE('',*,*,#2757,.T.);
#3561=ORIENTED_EDGE('',*,*,#2758,.T.);
#3562=ORIENTED_EDGE('',*,*,#2759,.F.);
#3563=ORIENTED_EDGE('',*,*,#2760,.T.);
#3564=ORIENTED_EDGE('',*,*,#2761,.T.);
#3565=ORIENTED_EDGE('',*,*,#2762,.T.);
#3566=ORIENTED_EDGE('',*,*,#2763,.F.);
#3567=ORIENTED_EDGE('',*,*,#2764,.T.);
#3568=ORIENTED_EDGE('',*,*,#2765,.T.);
#3569=ORIENTED_EDGE('',*,*,#2766,.T.);
#3570=ORIENTED_EDGE('',*,*,#2767,.F.);
#3571=ORIENTED_EDGE('',*,*,#2768,.T.);
#3572=ORIENTED_EDGE('',*,*,#2769,.T.);
#3573=ORIENTED_EDGE('',*,*,#2770,.F.);
#3574=ORIENTED_EDGE('',*,*,#2771,.T.);
#3575=ORIENTED_EDGE('',*,*,#2772,.F.);
#3576=ORIENTED_EDGE('',*,*,#2773,.F.);
#3577=ORIENTED_EDGE('',*,*,#2774,.T.);
#3578=ORIENTED_EDGE('',*,*,#2775,.F.);
#3579=ORIENTED_EDGE('',*,*,#2776,.T.);
#3580=ORIENTED_EDGE('',*,*,#2777,.T.);
#3581=ORIENTED_EDGE('',*,*,#2778,.F.);
#3582=ORIENTED_EDGE('',*,*,#2779,.F.);
#3583=ORIENTED_EDGE('',*,*,#2780,.T.);
#3584=ORIENTED_EDGE('',*,*,#2781,.T.);
#3585=ORIENTED_EDGE('',*,*,#2782,.F.);
#3586=ORIENTED_EDGE('',*,*,#2783,.F.);
#3587=ORIENTED_EDGE('',*,*,#2784,.T.);
#3588=ORIENTED_EDGE('',*,*,#2785,.T.);
#3589=ORIENTED_EDGE('',*,*,#2786,.F.);
#3590=ORIENTED_EDGE('',*,*,#2787,.F.);
#3591=ORIENTED_EDGE('',*,*,#2788,.F.);
#3592=ORIENTED_EDGE('',*,*,#2789,.T.);
#3593=ORIENTED_EDGE('',*,*,#2790,.T.);
#3594=ORIENTED_EDGE('',*,*,#2791,.F.);
#3595=ORIENTED_EDGE('',*,*,#2792,.T.);
#3596=ORIENTED_EDGE('',*,*,#2793,.F.);
#3597=ORIENTED_EDGE('',*,*,#2794,.T.);
#3598=ORIENTED_EDGE('',*,*,#2795,.T.);
#3599=ORIENTED_EDGE('',*,*,#2796,.F.);
#3600=ORIENTED_EDGE('',*,*,#2797,.F.);
#3601=ORIENTED_EDGE('',*,*,#2798,.F.);
#3602=ORIENTED_EDGE('',*,*,#2769,.F.);
#3603=ORIENTED_EDGE('',*,*,#2799,.T.);
#3604=ORIENTED_EDGE('',*,*,#2772,.T.);
#3605=ORIENTED_EDGE('',*,*,#2800,.F.);
#3606=ORIENTED_EDGE('',*,*,#2801,.F.);
#3607=ORIENTED_EDGE('',*,*,#2802,.T.);
#3608=ORIENTED_EDGE('',*,*,#2775,.T.);
#3609=ORIENTED_EDGE('',*,*,#2803,.F.);
#3610=ORIENTED_EDGE('',*,*,#2790,.F.);
#3611=ORIENTED_EDGE('',*,*,#2804,.T.);
#3612=ORIENTED_EDGE('',*,*,#2793,.T.);
#3613=ORIENTED_EDGE('',*,*,#2805,.F.);
#3614=ORIENTED_EDGE('',*,*,#2806,.T.);
#3615=ORIENTED_EDGE('',*,*,#2807,.F.);
#3616=ORIENTED_EDGE('',*,*,#2797,.T.);
#3617=ORIENTED_EDGE('',*,*,#2808,.T.);
#3618=ORIENTED_EDGE('',*,*,#2809,.T.);
#3619=ORIENTED_EDGE('',*,*,#2810,.F.);
#3620=ORIENTED_EDGE('',*,*,#2787,.T.);
#3621=ORIENTED_EDGE('',*,*,#2811,.T.);
#3622=ORIENTED_EDGE('',*,*,#2812,.T.);
#3623=ORIENTED_EDGE('',*,*,#2813,.F.);
#3624=ORIENTED_EDGE('',*,*,#2783,.T.);
#3625=ORIENTED_EDGE('',*,*,#2814,.T.);
#3626=ORIENTED_EDGE('',*,*,#2815,.T.);
#3627=ORIENTED_EDGE('',*,*,#2816,.F.);
#3628=ORIENTED_EDGE('',*,*,#2779,.T.);
#3629=ORIENTED_EDGE('',*,*,#2817,.T.);
#3630=ORIENTED_EDGE('',*,*,#2818,.F.);
#3631=ORIENTED_EDGE('',*,*,#2819,.T.);
#3632=ORIENTED_EDGE('',*,*,#2820,.F.);
#3633=ORIENTED_EDGE('',*,*,#2821,.T.);
#3634=ORIENTED_EDGE('',*,*,#2822,.T.);
#3635=ORIENTED_EDGE('',*,*,#2823,.F.);
#3636=ORIENTED_EDGE('',*,*,#2629,.T.);
#3637=ORIENTED_EDGE('',*,*,#2824,.F.);
#3638=ORIENTED_EDGE('',*,*,#2825,.T.);
#3639=ORIENTED_EDGE('',*,*,#2637,.F.);
#3640=ORIENTED_EDGE('',*,*,#2655,.T.);
#3641=ORIENTED_EDGE('',*,*,#2826,.T.);
#3642=ORIENTED_EDGE('',*,*,#2733,.F.);
#3643=ORIENTED_EDGE('',*,*,#2632,.F.);
#3644=ORIENTED_EDGE('',*,*,#2827,.F.);
#3645=ORIENTED_EDGE('',*,*,#2729,.F.);
#3646=ORIENTED_EDGE('',*,*,#2828,.F.);
#3647=ORIENTED_EDGE('',*,*,#2829,.F.);
#3648=ORIENTED_EDGE('',*,*,#2654,.F.);
#3649=ORIENTED_EDGE('',*,*,#2649,.T.);
#3650=ORIENTED_EDGE('',*,*,#2645,.F.);
#3651=ORIENTED_EDGE('',*,*,#2731,.F.);
#3652=ORIENTED_EDGE('',*,*,#2639,.T.);
#3653=ORIENTED_EDGE('',*,*,#2830,.T.);
#3654=ORIENTED_EDGE('',*,*,#2831,.F.);
#3655=ORIENTED_EDGE('',*,*,#2832,.F.);
#3656=ORIENTED_EDGE('',*,*,#2630,.T.);
#3657=ORIENTED_EDGE('',*,*,#2823,.T.);
#3658=ORIENTED_EDGE('',*,*,#2833,.T.);
#3659=ORIENTED_EDGE('',*,*,#2834,.F.);
#3660=ORIENTED_EDGE('',*,*,#2835,.T.);
#3661=ORIENTED_EDGE('',*,*,#2836,.T.);
#3662=ORIENTED_EDGE('',*,*,#2805,.T.);
#3663=ORIENTED_EDGE('',*,*,#2837,.F.);
#3664=ORIENTED_EDGE('',*,*,#2837,.T.);
#3665=ORIENTED_EDGE('',*,*,#2820,.T.);
#3666=ORIENTED_EDGE('',*,*,#2838,.F.);
#3667=ORIENTED_EDGE('',*,*,#2730,.F.);
#3668=ORIENTED_EDGE('',*,*,#2839,.F.);
#3669=ORIENTED_EDGE('',*,*,#2840,.F.);
#3670=ORIENTED_EDGE('',*,*,#2841,.F.);
#3671=ORIENTED_EDGE('',*,*,#2842,.F.);
#3672=ORIENTED_EDGE('',*,*,#2843,.F.);
#3673=ORIENTED_EDGE('',*,*,#2624,.T.);
#3674=ORIENTED_EDGE('',*,*,#2641,.F.);
#3675=ORIENTED_EDGE('',*,*,#2732,.T.);
#3676=ORIENTED_EDGE('',*,*,#2647,.T.);
#3677=ORIENTED_EDGE('',*,*,#2651,.F.);
#3678=ORIENTED_EDGE('',*,*,#2653,.F.);
#3679=ORIENTED_EDGE('',*,*,#2844,.T.);
#3680=ORIENTED_EDGE('',*,*,#2845,.F.);
#3681=ORIENTED_EDGE('',*,*,#2719,.T.);
#3682=ORIENTED_EDGE('',*,*,#2838,.T.);
#3683=ORIENTED_EDGE('',*,*,#2819,.F.);
#3684=ORIENTED_EDGE('',*,*,#2846,.F.);
#3685=ORIENTED_EDGE('',*,*,#2847,.F.);
#3686=ORIENTED_EDGE('',*,*,#2848,.T.);
#3687=ORIENTED_EDGE('',*,*,#2849,.T.);
#3688=ORIENTED_EDGE('',*,*,#2821,.F.);
#3689=ORIENTED_EDGE('',*,*,#2628,.F.);
#3690=ORIENTED_EDGE('',*,*,#2620,.T.);
#3691=ORIENTED_EDGE('',*,*,#2627,.T.);
#3692=ORIENTED_EDGE('',*,*,#2734,.F.);
#3693=ORIENTED_EDGE('',*,*,#2826,.F.);
#3694=ORIENTED_EDGE('',*,*,#2656,.T.);
#3695=ORIENTED_EDGE('',*,*,#2643,.T.);
#3696=ORIENTED_EDGE('',*,*,#2850,.F.);
#3697=ORIENTED_EDGE('',*,*,#2851,.F.);
#3698=ORIENTED_EDGE('',*,*,#2852,.F.);
#3699=ORIENTED_EDGE('',*,*,#2853,.F.);
#3700=ORIENTED_EDGE('',*,*,#2854,.F.);
#3701=ORIENTED_EDGE('',*,*,#2855,.T.);
#3702=ORIENTED_EDGE('',*,*,#2830,.F.);
#3703=ORIENTED_EDGE('',*,*,#2638,.F.);
#3704=ORIENTED_EDGE('',*,*,#2825,.F.);
#3705=ORIENTED_EDGE('',*,*,#2827,.T.);
#3706=ORIENTED_EDGE('',*,*,#2631,.T.);
#3707=ORIENTED_EDGE('',*,*,#2832,.T.);
#3708=ORIENTED_EDGE('',*,*,#2856,.F.);
#3709=ORIENTED_EDGE('',*,*,#2824,.T.);
#3710=ORIENTED_EDGE('',*,*,#2856,.T.);
#3711=ORIENTED_EDGE('',*,*,#2831,.T.);
#3712=ORIENTED_EDGE('',*,*,#2855,.F.);
#3713=ORIENTED_EDGE('',*,*,#2854,.T.);
#3714=ORIENTED_EDGE('',*,*,#2857,.T.);
#3715=ORIENTED_EDGE('',*,*,#2843,.T.);
#3716=ORIENTED_EDGE('',*,*,#2857,.F.);
#3717=ORIENTED_EDGE('',*,*,#2853,.T.);
#3718=ORIENTED_EDGE('',*,*,#2858,.T.);
#3719=ORIENTED_EDGE('',*,*,#2842,.T.);
#3720=ORIENTED_EDGE('',*,*,#2858,.F.);
#3721=ORIENTED_EDGE('',*,*,#2852,.T.);
#3722=ORIENTED_EDGE('',*,*,#2859,.T.);
#3723=ORIENTED_EDGE('',*,*,#2841,.T.);
#3724=ORIENTED_EDGE('',*,*,#2859,.F.);
#3725=ORIENTED_EDGE('',*,*,#2851,.T.);
#3726=ORIENTED_EDGE('',*,*,#2860,.T.);
#3727=ORIENTED_EDGE('',*,*,#2840,.T.);
#3728=ORIENTED_EDGE('',*,*,#2860,.F.);
#3729=ORIENTED_EDGE('',*,*,#2850,.T.);
#3730=ORIENTED_EDGE('',*,*,#2861,.T.);
#3731=ORIENTED_EDGE('',*,*,#2839,.T.);
#3732=ORIENTED_EDGE('',*,*,#2861,.F.);
#3733=ORIENTED_EDGE('',*,*,#2834,.T.);
#3734=ORIENTED_EDGE('',*,*,#2862,.T.);
#3735=ORIENTED_EDGE('',*,*,#2848,.F.);
#3736=ORIENTED_EDGE('',*,*,#2863,.F.);
#3737=ORIENTED_EDGE('',*,*,#2864,.F.);
#3738=ORIENTED_EDGE('',*,*,#2865,.T.);
#3739=ORIENTED_EDGE('',*,*,#2801,.T.);
#3740=ORIENTED_EDGE('',*,*,#2866,.F.);
#3741=ORIENTED_EDGE('',*,*,#2776,.F.);
#3742=ORIENTED_EDGE('',*,*,#2816,.T.);
#3743=ORIENTED_EDGE('',*,*,#2778,.T.);
#3744=ORIENTED_EDGE('',*,*,#2867,.T.);
#3745=ORIENTED_EDGE('',*,*,#2817,.F.);
#3746=ORIENTED_EDGE('',*,*,#2868,.F.);
#3747=ORIENTED_EDGE('',*,*,#2780,.F.);
#3748=ORIENTED_EDGE('',*,*,#2813,.T.);
#3749=ORIENTED_EDGE('',*,*,#2782,.T.);
#3750=ORIENTED_EDGE('',*,*,#2869,.T.);
#3751=ORIENTED_EDGE('',*,*,#2814,.F.);
#3752=ORIENTED_EDGE('',*,*,#2870,.F.);
#3753=ORIENTED_EDGE('',*,*,#2871,.F.);
#3754=ORIENTED_EDGE('',*,*,#2872,.T.);
#3755=ORIENTED_EDGE('',*,*,#2871,.T.);
#3756=ORIENTED_EDGE('',*,*,#2873,.T.);
#3757=ORIENTED_EDGE('',*,*,#2874,.F.);
#3758=ORIENTED_EDGE('',*,*,#2875,.F.);
#3759=ORIENTED_EDGE('',*,*,#2874,.T.);
#3760=ORIENTED_EDGE('',*,*,#2876,.T.);
#3761=ORIENTED_EDGE('',*,*,#2877,.F.);
#3762=ORIENTED_EDGE('',*,*,#2878,.F.);
#3763=ORIENTED_EDGE('',*,*,#2784,.F.);
#3764=ORIENTED_EDGE('',*,*,#2810,.T.);
#3765=ORIENTED_EDGE('',*,*,#2786,.T.);
#3766=ORIENTED_EDGE('',*,*,#2879,.T.);
#3767=ORIENTED_EDGE('',*,*,#2811,.F.);
#3768=ORIENTED_EDGE('',*,*,#2880,.F.);
#3769=ORIENTED_EDGE('',*,*,#2794,.F.);
#3770=ORIENTED_EDGE('',*,*,#2807,.T.);
#3771=ORIENTED_EDGE('',*,*,#2796,.T.);
#3772=ORIENTED_EDGE('',*,*,#2881,.T.);
#3773=ORIENTED_EDGE('',*,*,#2808,.F.);
#3774=ORIENTED_EDGE('',*,*,#2882,.F.);
#3775=ORIENTED_EDGE('',*,*,#2835,.F.);
#3776=ORIENTED_EDGE('',*,*,#2863,.T.);
#3777=ORIENTED_EDGE('',*,*,#2847,.T.);
#3778=ORIENTED_EDGE('',*,*,#2883,.F.);
#3779=ORIENTED_EDGE('',*,*,#2770,.T.);
#3780=ORIENTED_EDGE('',*,*,#2799,.F.);
#3781=ORIENTED_EDGE('',*,*,#2768,.F.);
#3782=ORIENTED_EDGE('',*,*,#2884,.F.);
#3783=ORIENTED_EDGE('',*,*,#2773,.T.);
#3784=ORIENTED_EDGE('',*,*,#2802,.F.);
#3785=ORIENTED_EDGE('',*,*,#2865,.F.);
#3786=ORIENTED_EDGE('',*,*,#2885,.F.);
#3787=ORIENTED_EDGE('',*,*,#2872,.F.);
#3788=ORIENTED_EDGE('',*,*,#2875,.T.);
#3789=ORIENTED_EDGE('',*,*,#2877,.T.);
#3790=ORIENTED_EDGE('',*,*,#2886,.F.);
#3791=ORIENTED_EDGE('',*,*,#2791,.T.);
#3792=ORIENTED_EDGE('',*,*,#2804,.F.);
#3793=ORIENTED_EDGE('',*,*,#2789,.F.);
#3794=ORIENTED_EDGE('',*,*,#2882,.T.);
#3795=ORIENTED_EDGE('',*,*,#2788,.T.);
#3796=ORIENTED_EDGE('',*,*,#2803,.T.);
#3797=ORIENTED_EDGE('',*,*,#2792,.F.);
#3798=ORIENTED_EDGE('',*,*,#2886,.T.);
#3799=ORIENTED_EDGE('',*,*,#2876,.F.);
#3800=ORIENTED_EDGE('',*,*,#2873,.F.);
#3801=ORIENTED_EDGE('',*,*,#2870,.T.);
#3802=ORIENTED_EDGE('',*,*,#2885,.T.);
#3803=ORIENTED_EDGE('',*,*,#2864,.T.);
#3804=ORIENTED_EDGE('',*,*,#2800,.T.);
#3805=ORIENTED_EDGE('',*,*,#2774,.F.);
#3806=ORIENTED_EDGE('',*,*,#2884,.T.);
#3807=ORIENTED_EDGE('',*,*,#2767,.T.);
#3808=ORIENTED_EDGE('',*,*,#2798,.T.);
#3809=ORIENTED_EDGE('',*,*,#2771,.F.);
#3810=ORIENTED_EDGE('',*,*,#2883,.T.);
#3811=ORIENTED_EDGE('',*,*,#2846,.T.);
#3812=ORIENTED_EDGE('',*,*,#2818,.T.);
#3813=ORIENTED_EDGE('',*,*,#2867,.F.);
#3814=ORIENTED_EDGE('',*,*,#2777,.F.);
#3815=ORIENTED_EDGE('',*,*,#2866,.T.);
#3816=ORIENTED_EDGE('',*,*,#2815,.F.);
#3817=ORIENTED_EDGE('',*,*,#2869,.F.);
#3818=ORIENTED_EDGE('',*,*,#2781,.F.);
#3819=ORIENTED_EDGE('',*,*,#2868,.T.);
#3820=ORIENTED_EDGE('',*,*,#2812,.F.);
#3821=ORIENTED_EDGE('',*,*,#2879,.F.);
#3822=ORIENTED_EDGE('',*,*,#2785,.F.);
#3823=ORIENTED_EDGE('',*,*,#2878,.T.);
#3824=ORIENTED_EDGE('',*,*,#2809,.F.);
#3825=ORIENTED_EDGE('',*,*,#2881,.F.);
#3826=ORIENTED_EDGE('',*,*,#2795,.F.);
#3827=ORIENTED_EDGE('',*,*,#2880,.T.);
#3828=ORIENTED_EDGE('',*,*,#2806,.F.);
#3829=ORIENTED_EDGE('',*,*,#2836,.F.);
#3830=ORIENTED_EDGE('',*,*,#2887,.T.);
#3831=ORIENTED_EDGE('',*,*,#2888,.T.);
#3832=ORIENTED_EDGE('',*,*,#2889,.F.);
#3833=ORIENTED_EDGE('',*,*,#2890,.T.);
#3834=ORIENTED_EDGE('',*,*,#2891,.T.);
#3835=ORIENTED_EDGE('',*,*,#2892,.T.);
#3836=ORIENTED_EDGE('',*,*,#2893,.F.);
#3837=ORIENTED_EDGE('',*,*,#2894,.T.);
#3838=ORIENTED_EDGE('',*,*,#2895,.T.);
#3839=ORIENTED_EDGE('',*,*,#2896,.T.);
#3840=ORIENTED_EDGE('',*,*,#2897,.F.);
#3841=ORIENTED_EDGE('',*,*,#2898,.F.);
#3842=ORIENTED_EDGE('',*,*,#2899,.T.);
#3843=ORIENTED_EDGE('',*,*,#2900,.T.);
#3844=ORIENTED_EDGE('',*,*,#2901,.F.);
#3845=ORIENTED_EDGE('',*,*,#2902,.F.);
#3846=ORIENTED_EDGE('',*,*,#2903,.T.);
#3847=ORIENTED_EDGE('',*,*,#2904,.T.);
#3848=ORIENTED_EDGE('',*,*,#2905,.F.);
#3849=ORIENTED_EDGE('',*,*,#2906,.F.);
#3850=ORIENTED_EDGE('',*,*,#2907,.T.);
#3851=ORIENTED_EDGE('',*,*,#2908,.T.);
#3852=ORIENTED_EDGE('',*,*,#2909,.F.);
#3853=ORIENTED_EDGE('',*,*,#2910,.F.);
#3854=ORIENTED_EDGE('',*,*,#2911,.T.);
#3855=ORIENTED_EDGE('',*,*,#2912,.T.);
#3856=ORIENTED_EDGE('',*,*,#2913,.F.);
#3857=ORIENTED_EDGE('',*,*,#2914,.T.);
#3858=ORIENTED_EDGE('',*,*,#2915,.T.);
#3859=ORIENTED_EDGE('',*,*,#2916,.T.);
#3860=ORIENTED_EDGE('',*,*,#2917,.F.);
#3861=ORIENTED_EDGE('',*,*,#2918,.F.);
#3862=ORIENTED_EDGE('',*,*,#2919,.T.);
#3863=ORIENTED_EDGE('',*,*,#2920,.T.);
#3864=ORIENTED_EDGE('',*,*,#2918,.T.);
#3865=ORIENTED_EDGE('',*,*,#2921,.T.);
#3866=ORIENTED_EDGE('',*,*,#2737,.F.);
#3867=ORIENTED_EDGE('',*,*,#2921,.F.);
#3868=ORIENTED_EDGE('',*,*,#2917,.T.);
#3869=ORIENTED_EDGE('',*,*,#2922,.T.);
#3870=ORIENTED_EDGE('',*,*,#2738,.F.);
#3871=ORIENTED_EDGE('',*,*,#2916,.F.);
#3872=ORIENTED_EDGE('',*,*,#2923,.T.);
#3873=ORIENTED_EDGE('',*,*,#2924,.T.);
#3874=ORIENTED_EDGE('',*,*,#2735,.T.);
#3875=ORIENTED_EDGE('',*,*,#2922,.F.);
#3876=ORIENTED_EDGE('',*,*,#2914,.F.);
#3877=ORIENTED_EDGE('',*,*,#2925,.T.);
#3878=ORIENTED_EDGE('',*,*,#2741,.T.);
#3879=ORIENTED_EDGE('',*,*,#2926,.F.);
#3880=ORIENTED_EDGE('',*,*,#2925,.F.);
#3881=ORIENTED_EDGE('',*,*,#2913,.T.);
#3882=ORIENTED_EDGE('',*,*,#2927,.T.);
#3883=ORIENTED_EDGE('',*,*,#2928,.T.);
#3884=ORIENTED_EDGE('',*,*,#2742,.F.);
#3885=ORIENTED_EDGE('',*,*,#2911,.F.);
#3886=ORIENTED_EDGE('',*,*,#2926,.T.);
#3887=ORIENTED_EDGE('',*,*,#2740,.T.);
#3888=ORIENTED_EDGE('',*,*,#2929,.T.);
#3889=ORIENTED_EDGE('',*,*,#2930,.T.);
#3890=ORIENTED_EDGE('',*,*,#2931,.T.);
#3891=ORIENTED_EDGE('',*,*,#2932,.T.);
#3892=ORIENTED_EDGE('',*,*,#2910,.T.);
#3893=ORIENTED_EDGE('',*,*,#2933,.T.);
#3894=ORIENTED_EDGE('',*,*,#2765,.F.);
#3895=ORIENTED_EDGE('',*,*,#2933,.F.);
#3896=ORIENTED_EDGE('',*,*,#2909,.T.);
#3897=ORIENTED_EDGE('',*,*,#2934,.T.);
#3898=ORIENTED_EDGE('',*,*,#2766,.F.);
#3899=ORIENTED_EDGE('',*,*,#2908,.F.);
#3900=ORIENTED_EDGE('',*,*,#2935,.T.);
#3901=ORIENTED_EDGE('',*,*,#2936,.T.);
#3902=ORIENTED_EDGE('',*,*,#2763,.T.);
#3903=ORIENTED_EDGE('',*,*,#2934,.F.);
#3904=ORIENTED_EDGE('',*,*,#2937,.T.);
#3905=ORIENTED_EDGE('',*,*,#2938,.T.);
#3906=ORIENTED_EDGE('',*,*,#2906,.T.);
#3907=ORIENTED_EDGE('',*,*,#2939,.T.);
#3908=ORIENTED_EDGE('',*,*,#2745,.F.);
#3909=ORIENTED_EDGE('',*,*,#2939,.F.);
#3910=ORIENTED_EDGE('',*,*,#2905,.T.);
#3911=ORIENTED_EDGE('',*,*,#2940,.T.);
#3912=ORIENTED_EDGE('',*,*,#2746,.F.);
#3913=ORIENTED_EDGE('',*,*,#2904,.F.);
#3914=ORIENTED_EDGE('',*,*,#2941,.T.);
#3915=ORIENTED_EDGE('',*,*,#2942,.T.);
#3916=ORIENTED_EDGE('',*,*,#2743,.T.);
#3917=ORIENTED_EDGE('',*,*,#2940,.F.);
#3918=ORIENTED_EDGE('',*,*,#2943,.T.);
#3919=ORIENTED_EDGE('',*,*,#2944,.T.);
#3920=ORIENTED_EDGE('',*,*,#2902,.T.);
#3921=ORIENTED_EDGE('',*,*,#2945,.T.);
#3922=ORIENTED_EDGE('',*,*,#2761,.F.);
#3923=ORIENTED_EDGE('',*,*,#2945,.F.);
#3924=ORIENTED_EDGE('',*,*,#2901,.T.);
#3925=ORIENTED_EDGE('',*,*,#2946,.T.);
#3926=ORIENTED_EDGE('',*,*,#2762,.F.);
#3927=ORIENTED_EDGE('',*,*,#2900,.F.);
#3928=ORIENTED_EDGE('',*,*,#2947,.T.);
#3929=ORIENTED_EDGE('',*,*,#2948,.T.);
#3930=ORIENTED_EDGE('',*,*,#2759,.T.);
#3931=ORIENTED_EDGE('',*,*,#2946,.F.);
#3932=ORIENTED_EDGE('',*,*,#2949,.T.);
#3933=ORIENTED_EDGE('',*,*,#2950,.T.);
#3934=ORIENTED_EDGE('',*,*,#2898,.T.);
#3935=ORIENTED_EDGE('',*,*,#2951,.T.);
#3936=ORIENTED_EDGE('',*,*,#2757,.F.);
#3937=ORIENTED_EDGE('',*,*,#2951,.F.);
#3938=ORIENTED_EDGE('',*,*,#2897,.T.);
#3939=ORIENTED_EDGE('',*,*,#2952,.T.);
#3940=ORIENTED_EDGE('',*,*,#2758,.F.);
#3941=ORIENTED_EDGE('',*,*,#2896,.F.);
#3942=ORIENTED_EDGE('',*,*,#2953,.T.);
#3943=ORIENTED_EDGE('',*,*,#2954,.T.);
#3944=ORIENTED_EDGE('',*,*,#2755,.T.);
#3945=ORIENTED_EDGE('',*,*,#2952,.F.);
#3946=ORIENTED_EDGE('',*,*,#2894,.F.);
#3947=ORIENTED_EDGE('',*,*,#2955,.T.);
#3948=ORIENTED_EDGE('',*,*,#2749,.T.);
#3949=ORIENTED_EDGE('',*,*,#2956,.F.);
#3950=ORIENTED_EDGE('',*,*,#2955,.F.);
#3951=ORIENTED_EDGE('',*,*,#2893,.T.);
#3952=ORIENTED_EDGE('',*,*,#2957,.T.);
#3953=ORIENTED_EDGE('',*,*,#2958,.T.);
#3954=ORIENTED_EDGE('',*,*,#2750,.F.);
#3955=ORIENTED_EDGE('',*,*,#2891,.F.);
#3956=ORIENTED_EDGE('',*,*,#2956,.T.);
#3957=ORIENTED_EDGE('',*,*,#2748,.T.);
#3958=ORIENTED_EDGE('',*,*,#2959,.T.);
#3959=ORIENTED_EDGE('',*,*,#2960,.T.);
#3960=ORIENTED_EDGE('',*,*,#2890,.F.);
#3961=ORIENTED_EDGE('',*,*,#2961,.T.);
#3962=ORIENTED_EDGE('',*,*,#2753,.T.);
#3963=ORIENTED_EDGE('',*,*,#2962,.F.);
#3964=ORIENTED_EDGE('',*,*,#2961,.F.);
#3965=ORIENTED_EDGE('',*,*,#2889,.T.);
#3966=ORIENTED_EDGE('',*,*,#2963,.T.);
#3967=ORIENTED_EDGE('',*,*,#2964,.T.);
#3968=ORIENTED_EDGE('',*,*,#2754,.F.);
#3969=ORIENTED_EDGE('',*,*,#2887,.F.);
#3970=ORIENTED_EDGE('',*,*,#2962,.T.);
#3971=ORIENTED_EDGE('',*,*,#2752,.T.);
#3972=ORIENTED_EDGE('',*,*,#2965,.T.);
#3973=ORIENTED_EDGE('',*,*,#2966,.T.);
#3974=ORIENTED_EDGE('',*,*,#2907,.F.);
#3975=ORIENTED_EDGE('',*,*,#2932,.F.);
#3976=ORIENTED_EDGE('',*,*,#2967,.F.);
#3977=ORIENTED_EDGE('',*,*,#2935,.F.);
#3978=ORIENTED_EDGE('',*,*,#2931,.F.);
#3979=ORIENTED_EDGE('',*,*,#2764,.F.);
#3980=ORIENTED_EDGE('',*,*,#2936,.F.);
#3981=ORIENTED_EDGE('',*,*,#2967,.T.);
#3982=ORIENTED_EDGE('',*,*,#2899,.F.);
#3983=ORIENTED_EDGE('',*,*,#2944,.F.);
#3984=ORIENTED_EDGE('',*,*,#2968,.F.);
#3985=ORIENTED_EDGE('',*,*,#2947,.F.);
#3986=ORIENTED_EDGE('',*,*,#2943,.F.);
#3987=ORIENTED_EDGE('',*,*,#2760,.F.);
#3988=ORIENTED_EDGE('',*,*,#2948,.F.);
#3989=ORIENTED_EDGE('',*,*,#2968,.T.);
#3990=ORIENTED_EDGE('',*,*,#2895,.F.);
#3991=ORIENTED_EDGE('',*,*,#2950,.F.);
#3992=ORIENTED_EDGE('',*,*,#2969,.F.);
#3993=ORIENTED_EDGE('',*,*,#2953,.F.);
#3994=ORIENTED_EDGE('',*,*,#2949,.F.);
#3995=ORIENTED_EDGE('',*,*,#2756,.F.);
#3996=ORIENTED_EDGE('',*,*,#2954,.F.);
#3997=ORIENTED_EDGE('',*,*,#2969,.T.);
#3998=ORIENTED_EDGE('',*,*,#2970,.F.);
#3999=ORIENTED_EDGE('',*,*,#2963,.F.);
#4000=ORIENTED_EDGE('',*,*,#2888,.F.);
#4001=ORIENTED_EDGE('',*,*,#2966,.F.);
#4002=ORIENTED_EDGE('',*,*,#2964,.F.);
#4003=ORIENTED_EDGE('',*,*,#2970,.T.);
#4004=ORIENTED_EDGE('',*,*,#2965,.F.);
#4005=ORIENTED_EDGE('',*,*,#2751,.F.);
#4006=ORIENTED_EDGE('',*,*,#2971,.F.);
#4007=ORIENTED_EDGE('',*,*,#2957,.F.);
#4008=ORIENTED_EDGE('',*,*,#2892,.F.);
#4009=ORIENTED_EDGE('',*,*,#2960,.F.);
#4010=ORIENTED_EDGE('',*,*,#2958,.F.);
#4011=ORIENTED_EDGE('',*,*,#2971,.T.);
#4012=ORIENTED_EDGE('',*,*,#2959,.F.);
#4013=ORIENTED_EDGE('',*,*,#2747,.F.);
#4014=ORIENTED_EDGE('',*,*,#2903,.F.);
#4015=ORIENTED_EDGE('',*,*,#2938,.F.);
#4016=ORIENTED_EDGE('',*,*,#2972,.F.);
#4017=ORIENTED_EDGE('',*,*,#2941,.F.);
#4018=ORIENTED_EDGE('',*,*,#2937,.F.);
#4019=ORIENTED_EDGE('',*,*,#2744,.F.);
#4020=ORIENTED_EDGE('',*,*,#2942,.F.);
#4021=ORIENTED_EDGE('',*,*,#2972,.T.);
#4022=ORIENTED_EDGE('',*,*,#2973,.F.);
#4023=ORIENTED_EDGE('',*,*,#2927,.F.);
#4024=ORIENTED_EDGE('',*,*,#2912,.F.);
#4025=ORIENTED_EDGE('',*,*,#2930,.F.);
#4026=ORIENTED_EDGE('',*,*,#2928,.F.);
#4027=ORIENTED_EDGE('',*,*,#2973,.T.);
#4028=ORIENTED_EDGE('',*,*,#2929,.F.);
#4029=ORIENTED_EDGE('',*,*,#2739,.F.);
#4030=ORIENTED_EDGE('',*,*,#2915,.F.);
#4031=ORIENTED_EDGE('',*,*,#2920,.F.);
#4032=ORIENTED_EDGE('',*,*,#2974,.F.);
#4033=ORIENTED_EDGE('',*,*,#2923,.F.);
#4034=ORIENTED_EDGE('',*,*,#2919,.F.);
#4035=ORIENTED_EDGE('',*,*,#2736,.F.);
#4036=ORIENTED_EDGE('',*,*,#2924,.F.);
#4037=ORIENTED_EDGE('',*,*,#2974,.T.);
#4038=ORIENTED_EDGE('',*,*,#2975,.F.);
#4039=ORIENTED_EDGE('',*,*,#2976,.F.);
#4040=ORIENTED_EDGE('',*,*,#2977,.T.);
#4041=ORIENTED_EDGE('',*,*,#2976,.T.);
#4042=ORIENTED_EDGE('',*,*,#2978,.T.);
#4043=ORIENTED_EDGE('',*,*,#2979,.F.);
#4044=ORIENTED_EDGE('',*,*,#2980,.F.);
#4045=ORIENTED_EDGE('',*,*,#2979,.T.);
#4046=ORIENTED_EDGE('',*,*,#2981,.T.);
#4047=ORIENTED_EDGE('',*,*,#2982,.F.);
#4048=ORIENTED_EDGE('',*,*,#2702,.T.);
#4049=ORIENTED_EDGE('',*,*,#2983,.T.);
#4050=ORIENTED_EDGE('',*,*,#2984,.F.);
#4051=ORIENTED_EDGE('',*,*,#2985,.F.);
#4052=ORIENTED_EDGE('',*,*,#2984,.T.);
#4053=ORIENTED_EDGE('',*,*,#2986,.T.);
#4054=ORIENTED_EDGE('',*,*,#2987,.F.);
#4055=ORIENTED_EDGE('',*,*,#2708,.T.);
#4056=ORIENTED_EDGE('',*,*,#2988,.T.);
#4057=ORIENTED_EDGE('',*,*,#2725,.F.);
#4058=ORIENTED_EDGE('',*,*,#2989,.F.);
#4059=ORIENTED_EDGE('',*,*,#2990,.F.);
#4060=ORIENTED_EDGE('',*,*,#2991,.T.);
#4061=ORIENTED_EDGE('',*,*,#2990,.T.);
#4062=ORIENTED_EDGE('',*,*,#2992,.T.);
#4063=ORIENTED_EDGE('',*,*,#2710,.F.);
#4064=ORIENTED_EDGE('',*,*,#2993,.F.);
#4065=ORIENTED_EDGE('',*,*,#2994,.F.);
#4066=ORIENTED_EDGE('',*,*,#2995,.F.);
#4067=ORIENTED_EDGE('',*,*,#2996,.T.);
#4068=ORIENTED_EDGE('',*,*,#2995,.T.);
#4069=ORIENTED_EDGE('',*,*,#2997,.T.);
#4070=ORIENTED_EDGE('',*,*,#2998,.F.);
#4071=ORIENTED_EDGE('',*,*,#2999,.F.);
#4072=ORIENTED_EDGE('',*,*,#2998,.T.);
#4073=ORIENTED_EDGE('',*,*,#3000,.T.);
#4074=ORIENTED_EDGE('',*,*,#3001,.F.);
#4075=ORIENTED_EDGE('',*,*,#3002,.F.);
#4076=ORIENTED_EDGE('',*,*,#2697,.F.);
#4077=ORIENTED_EDGE('',*,*,#2723,.T.);
#4078=ORIENTED_EDGE('',*,*,#2700,.T.);
#4079=ORIENTED_EDGE('',*,*,#3003,.F.);
#4080=ORIENTED_EDGE('',*,*,#2715,.F.);
#4081=ORIENTED_EDGE('',*,*,#2727,.T.);
#4082=ORIENTED_EDGE('',*,*,#2718,.T.);
#4083=ORIENTED_EDGE('',*,*,#3004,.F.);
#4084=ORIENTED_EDGE('',*,*,#2691,.F.);
#4085=ORIENTED_EDGE('',*,*,#2721,.T.);
#4086=ORIENTED_EDGE('',*,*,#2694,.T.);
#4087=ORIENTED_EDGE('',*,*,#3005,.F.);
#4088=ORIENTED_EDGE('',*,*,#2844,.F.);
#4089=ORIENTED_EDGE('',*,*,#2652,.F.);
#4090=ORIENTED_EDGE('',*,*,#2829,.T.);
#4091=ORIENTED_EDGE('',*,*,#3006,.F.);
#4092=ORIENTED_EDGE('',*,*,#2996,.F.);
#4093=ORIENTED_EDGE('',*,*,#2999,.T.);
#4094=ORIENTED_EDGE('',*,*,#3001,.T.);
#4095=ORIENTED_EDGE('',*,*,#3007,.F.);
#4096=ORIENTED_EDGE('',*,*,#2991,.F.);
#4097=ORIENTED_EDGE('',*,*,#2993,.T.);
#4098=ORIENTED_EDGE('',*,*,#2712,.T.);
#4099=ORIENTED_EDGE('',*,*,#3008,.F.);
#4100=ORIENTED_EDGE('',*,*,#2703,.F.);
#4101=ORIENTED_EDGE('',*,*,#2985,.T.);
#4102=ORIENTED_EDGE('',*,*,#2987,.T.);
#4103=ORIENTED_EDGE('',*,*,#3009,.F.);
#4104=ORIENTED_EDGE('',*,*,#2977,.F.);
#4105=ORIENTED_EDGE('',*,*,#2980,.T.);
#4106=ORIENTED_EDGE('',*,*,#2982,.T.);
#4107=ORIENTED_EDGE('',*,*,#2845,.T.);
#4108=ORIENTED_EDGE('',*,*,#3005,.T.);
#4109=ORIENTED_EDGE('',*,*,#2981,.F.);
#4110=ORIENTED_EDGE('',*,*,#2978,.F.);
#4111=ORIENTED_EDGE('',*,*,#2975,.T.);
#4112=ORIENTED_EDGE('',*,*,#3009,.T.);
#4113=ORIENTED_EDGE('',*,*,#2986,.F.);
#4114=ORIENTED_EDGE('',*,*,#2983,.F.);
#4115=ORIENTED_EDGE('',*,*,#2701,.T.);
#4116=ORIENTED_EDGE('',*,*,#3008,.T.);
#4117=ORIENTED_EDGE('',*,*,#2711,.F.);
#4118=ORIENTED_EDGE('',*,*,#2992,.F.);
#4119=ORIENTED_EDGE('',*,*,#2989,.T.);
#4120=ORIENTED_EDGE('',*,*,#3007,.T.);
#4121=ORIENTED_EDGE('',*,*,#3000,.F.);
#4122=ORIENTED_EDGE('',*,*,#2997,.F.);
#4123=ORIENTED_EDGE('',*,*,#2994,.T.);
#4124=ORIENTED_EDGE('',*,*,#3006,.T.);
#4125=ORIENTED_EDGE('',*,*,#2828,.T.);
#4126=ORIENTED_EDGE('',*,*,#2728,.T.);
#4127=ORIENTED_EDGE('',*,*,#2713,.T.);
#4128=ORIENTED_EDGE('',*,*,#3003,.T.);
#4129=ORIENTED_EDGE('',*,*,#2717,.F.);
#4130=ORIENTED_EDGE('',*,*,#2726,.F.);
#4131=ORIENTED_EDGE('',*,*,#2988,.F.);
#4132=ORIENTED_EDGE('',*,*,#2707,.F.);
#4133=ORIENTED_EDGE('',*,*,#2704,.T.);
#4134=ORIENTED_EDGE('',*,*,#2724,.F.);
#4135=ORIENTED_EDGE('',*,*,#2695,.T.);
#4136=ORIENTED_EDGE('',*,*,#3002,.T.);
#4137=ORIENTED_EDGE('',*,*,#2699,.F.);
#4138=ORIENTED_EDGE('',*,*,#2722,.F.);
#4139=ORIENTED_EDGE('',*,*,#2689,.T.);
#4140=ORIENTED_EDGE('',*,*,#3004,.T.);
#4141=ORIENTED_EDGE('',*,*,#2693,.F.);
#4142=ORIENTED_EDGE('',*,*,#2720,.F.);
#4143=ORIENTED_EDGE('',*,*,#3010,.T.);
#4144=ORIENTED_EDGE('',*,*,#3011,.T.);
#4145=ORIENTED_EDGE('',*,*,#3012,.F.);
#4146=ORIENTED_EDGE('',*,*,#3013,.T.);
#4147=ORIENTED_EDGE('',*,*,#3014,.T.);
#4148=ORIENTED_EDGE('',*,*,#3015,.T.);
#4149=ORIENTED_EDGE('',*,*,#3016,.F.);
#4150=ORIENTED_EDGE('',*,*,#3017,.F.);
#4151=ORIENTED_EDGE('',*,*,#3018,.T.);
#4152=ORIENTED_EDGE('',*,*,#3019,.T.);
#4153=ORIENTED_EDGE('',*,*,#3020,.F.);
#4154=ORIENTED_EDGE('',*,*,#3021,.F.);
#4155=ORIENTED_EDGE('',*,*,#3022,.T.);
#4156=ORIENTED_EDGE('',*,*,#3023,.T.);
#4157=ORIENTED_EDGE('',*,*,#3024,.F.);
#4158=ORIENTED_EDGE('',*,*,#3025,.F.);
#4159=ORIENTED_EDGE('',*,*,#3026,.T.);
#4160=ORIENTED_EDGE('',*,*,#3027,.T.);
#4161=ORIENTED_EDGE('',*,*,#3028,.F.);
#4162=ORIENTED_EDGE('',*,*,#3029,.F.);
#4163=ORIENTED_EDGE('',*,*,#3030,.T.);
#4164=ORIENTED_EDGE('',*,*,#3031,.T.);
#4165=ORIENTED_EDGE('',*,*,#3032,.F.);
#4166=ORIENTED_EDGE('',*,*,#3033,.T.);
#4167=ORIENTED_EDGE('',*,*,#3034,.T.);
#4168=ORIENTED_EDGE('',*,*,#3035,.T.);
#4169=ORIENTED_EDGE('',*,*,#3036,.F.);
#4170=ORIENTED_EDGE('',*,*,#3037,.F.);
#4171=ORIENTED_EDGE('',*,*,#3038,.T.);
#4172=ORIENTED_EDGE('',*,*,#3039,.T.);
#4173=ORIENTED_EDGE('',*,*,#3040,.F.);
#4174=ORIENTED_EDGE('',*,*,#3041,.T.);
#4175=ORIENTED_EDGE('',*,*,#3041,.F.);
#4176=ORIENTED_EDGE('',*,*,#3042,.T.);
#4177=ORIENTED_EDGE('',*,*,#2680,.F.);
#4178=ORIENTED_EDGE('',*,*,#3043,.F.);
#4179=ORIENTED_EDGE('',*,*,#3042,.F.);
#4180=ORIENTED_EDGE('',*,*,#3040,.T.);
#4181=ORIENTED_EDGE('',*,*,#3044,.T.);
#4182=ORIENTED_EDGE('',*,*,#3045,.T.);
#4183=ORIENTED_EDGE('',*,*,#3046,.T.);
#4184=ORIENTED_EDGE('',*,*,#2677,.T.);
#4185=ORIENTED_EDGE('',*,*,#3047,.T.);
#4186=ORIENTED_EDGE('',*,*,#3048,.T.);
#4187=ORIENTED_EDGE('',*,*,#3045,.F.);
#4188=ORIENTED_EDGE('',*,*,#3049,.T.);
#4189=ORIENTED_EDGE('',*,*,#3038,.F.);
#4190=ORIENTED_EDGE('',*,*,#3043,.T.);
#4191=ORIENTED_EDGE('',*,*,#2679,.F.);
#4192=ORIENTED_EDGE('',*,*,#3050,.T.);
#4193=ORIENTED_EDGE('',*,*,#3047,.F.);
#4194=ORIENTED_EDGE('',*,*,#3051,.T.);
#4195=ORIENTED_EDGE('',*,*,#3052,.T.);
#4196=ORIENTED_EDGE('',*,*,#3053,.T.);
#4197=ORIENTED_EDGE('',*,*,#3054,.F.);
#4198=ORIENTED_EDGE('',*,*,#3055,.T.);
#4199=ORIENTED_EDGE('',*,*,#3052,.F.);
#4200=ORIENTED_EDGE('',*,*,#3056,.T.);
#4201=ORIENTED_EDGE('',*,*,#3037,.T.);
#4202=ORIENTED_EDGE('',*,*,#3057,.T.);
#4203=ORIENTED_EDGE('',*,*,#2686,.T.);
#4204=ORIENTED_EDGE('',*,*,#3058,.T.);
#4205=ORIENTED_EDGE('',*,*,#3057,.F.);
#4206=ORIENTED_EDGE('',*,*,#3036,.T.);
#4207=ORIENTED_EDGE('',*,*,#3059,.T.);
#4208=ORIENTED_EDGE('',*,*,#2687,.T.);
#4209=ORIENTED_EDGE('',*,*,#3035,.F.);
#4210=ORIENTED_EDGE('',*,*,#3060,.T.);
#4211=ORIENTED_EDGE('',*,*,#3054,.T.);
#4212=ORIENTED_EDGE('',*,*,#3061,.T.);
#4213=ORIENTED_EDGE('',*,*,#2688,.F.);
#4214=ORIENTED_EDGE('',*,*,#3059,.F.);
#4215=ORIENTED_EDGE('',*,*,#3033,.F.);
#4216=ORIENTED_EDGE('',*,*,#3062,.T.);
#4217=ORIENTED_EDGE('',*,*,#2660,.F.);
#4218=ORIENTED_EDGE('',*,*,#3063,.F.);
#4219=ORIENTED_EDGE('',*,*,#3062,.F.);
#4220=ORIENTED_EDGE('',*,*,#3032,.T.);
#4221=ORIENTED_EDGE('',*,*,#3064,.T.);
#4222=ORIENTED_EDGE('',*,*,#3065,.T.);
#4223=ORIENTED_EDGE('',*,*,#3066,.T.);
#4224=ORIENTED_EDGE('',*,*,#2657,.T.);
#4225=ORIENTED_EDGE('',*,*,#3067,.T.);
#4226=ORIENTED_EDGE('',*,*,#3068,.T.);
#4227=ORIENTED_EDGE('',*,*,#3065,.F.);
#4228=ORIENTED_EDGE('',*,*,#3069,.T.);
#4229=ORIENTED_EDGE('',*,*,#3030,.F.);
#4230=ORIENTED_EDGE('',*,*,#3063,.T.);
#4231=ORIENTED_EDGE('',*,*,#2659,.F.);
#4232=ORIENTED_EDGE('',*,*,#3070,.T.);
#4233=ORIENTED_EDGE('',*,*,#3067,.F.);
#4234=ORIENTED_EDGE('',*,*,#3071,.T.);
#4235=ORIENTED_EDGE('',*,*,#3072,.T.);
#4236=ORIENTED_EDGE('',*,*,#3073,.T.);
#4237=ORIENTED_EDGE('',*,*,#3074,.F.);
#4238=ORIENTED_EDGE('',*,*,#3075,.T.);
#4239=ORIENTED_EDGE('',*,*,#3072,.F.);
#4240=ORIENTED_EDGE('',*,*,#3076,.T.);
#4241=ORIENTED_EDGE('',*,*,#3029,.T.);
#4242=ORIENTED_EDGE('',*,*,#3077,.T.);
#4243=ORIENTED_EDGE('',*,*,#2670,.T.);
#4244=ORIENTED_EDGE('',*,*,#3078,.T.);
#4245=ORIENTED_EDGE('',*,*,#3077,.F.);
#4246=ORIENTED_EDGE('',*,*,#3028,.T.);
#4247=ORIENTED_EDGE('',*,*,#3079,.T.);
#4248=ORIENTED_EDGE('',*,*,#2671,.T.);
#4249=ORIENTED_EDGE('',*,*,#3027,.F.);
#4250=ORIENTED_EDGE('',*,*,#3080,.T.);
#4251=ORIENTED_EDGE('',*,*,#3074,.T.);
#4252=ORIENTED_EDGE('',*,*,#3081,.T.);
#4253=ORIENTED_EDGE('',*,*,#2672,.F.);
#4254=ORIENTED_EDGE('',*,*,#3079,.F.);
#4255=ORIENTED_EDGE('',*,*,#3082,.T.);
#4256=ORIENTED_EDGE('',*,*,#3083,.T.);
#4257=ORIENTED_EDGE('',*,*,#3084,.F.);
#4258=ORIENTED_EDGE('',*,*,#3085,.T.);
#4259=ORIENTED_EDGE('',*,*,#3082,.F.);
#4260=ORIENTED_EDGE('',*,*,#3086,.T.);
#4261=ORIENTED_EDGE('',*,*,#3025,.T.);
#4262=ORIENTED_EDGE('',*,*,#3087,.T.);
#4263=ORIENTED_EDGE('',*,*,#2682,.T.);
#4264=ORIENTED_EDGE('',*,*,#3088,.T.);
#4265=ORIENTED_EDGE('',*,*,#3087,.F.);
#4266=ORIENTED_EDGE('',*,*,#3024,.T.);
#4267=ORIENTED_EDGE('',*,*,#3089,.T.);
#4268=ORIENTED_EDGE('',*,*,#2683,.T.);
#4269=ORIENTED_EDGE('',*,*,#3023,.F.);
#4270=ORIENTED_EDGE('',*,*,#3090,.T.);
#4271=ORIENTED_EDGE('',*,*,#3084,.T.);
#4272=ORIENTED_EDGE('',*,*,#3091,.T.);
#4273=ORIENTED_EDGE('',*,*,#2684,.F.);
#4274=ORIENTED_EDGE('',*,*,#3089,.F.);
#4275=ORIENTED_EDGE('',*,*,#3092,.T.);
#4276=ORIENTED_EDGE('',*,*,#3093,.T.);
#4277=ORIENTED_EDGE('',*,*,#3094,.F.);
#4278=ORIENTED_EDGE('',*,*,#3095,.T.);
#4279=ORIENTED_EDGE('',*,*,#3092,.F.);
#4280=ORIENTED_EDGE('',*,*,#3096,.T.);
#4281=ORIENTED_EDGE('',*,*,#3021,.T.);
#4282=ORIENTED_EDGE('',*,*,#3097,.T.);
#4283=ORIENTED_EDGE('',*,*,#2674,.T.);
#4284=ORIENTED_EDGE('',*,*,#3098,.T.);
#4285=ORIENTED_EDGE('',*,*,#3097,.F.);
#4286=ORIENTED_EDGE('',*,*,#3020,.T.);
#4287=ORIENTED_EDGE('',*,*,#3099,.T.);
#4288=ORIENTED_EDGE('',*,*,#2675,.T.);
#4289=ORIENTED_EDGE('',*,*,#3019,.F.);
#4290=ORIENTED_EDGE('',*,*,#3100,.T.);
#4291=ORIENTED_EDGE('',*,*,#3094,.T.);
#4292=ORIENTED_EDGE('',*,*,#3101,.T.);
#4293=ORIENTED_EDGE('',*,*,#2676,.F.);
#4294=ORIENTED_EDGE('',*,*,#3099,.F.);
#4295=ORIENTED_EDGE('',*,*,#3102,.T.);
#4296=ORIENTED_EDGE('',*,*,#3103,.T.);
#4297=ORIENTED_EDGE('',*,*,#3104,.F.);
#4298=ORIENTED_EDGE('',*,*,#3105,.T.);
#4299=ORIENTED_EDGE('',*,*,#3102,.F.);
#4300=ORIENTED_EDGE('',*,*,#3106,.T.);
#4301=ORIENTED_EDGE('',*,*,#3017,.T.);
#4302=ORIENTED_EDGE('',*,*,#3107,.T.);
#4303=ORIENTED_EDGE('',*,*,#2666,.T.);
#4304=ORIENTED_EDGE('',*,*,#3108,.T.);
#4305=ORIENTED_EDGE('',*,*,#3107,.F.);
#4306=ORIENTED_EDGE('',*,*,#3016,.T.);
#4307=ORIENTED_EDGE('',*,*,#3109,.T.);
#4308=ORIENTED_EDGE('',*,*,#2667,.T.);
#4309=ORIENTED_EDGE('',*,*,#3015,.F.);
#4310=ORIENTED_EDGE('',*,*,#3110,.T.);
#4311=ORIENTED_EDGE('',*,*,#3104,.T.);
#4312=ORIENTED_EDGE('',*,*,#3111,.T.);
#4313=ORIENTED_EDGE('',*,*,#2668,.F.);
#4314=ORIENTED_EDGE('',*,*,#3109,.F.);
#4315=ORIENTED_EDGE('',*,*,#3013,.F.);
#4316=ORIENTED_EDGE('',*,*,#3112,.T.);
#4317=ORIENTED_EDGE('',*,*,#2664,.F.);
#4318=ORIENTED_EDGE('',*,*,#3113,.F.);
#4319=ORIENTED_EDGE('',*,*,#3112,.F.);
#4320=ORIENTED_EDGE('',*,*,#3012,.T.);
#4321=ORIENTED_EDGE('',*,*,#3114,.T.);
#4322=ORIENTED_EDGE('',*,*,#3115,.T.);
#4323=ORIENTED_EDGE('',*,*,#3116,.T.);
#4324=ORIENTED_EDGE('',*,*,#2661,.T.);
#4325=ORIENTED_EDGE('',*,*,#3117,.T.);
#4326=ORIENTED_EDGE('',*,*,#3118,.T.);
#4327=ORIENTED_EDGE('',*,*,#3115,.F.);
#4328=ORIENTED_EDGE('',*,*,#3119,.T.);
#4329=ORIENTED_EDGE('',*,*,#3010,.F.);
#4330=ORIENTED_EDGE('',*,*,#3113,.T.);
#4331=ORIENTED_EDGE('',*,*,#2663,.F.);
#4332=ORIENTED_EDGE('',*,*,#3120,.T.);
#4333=ORIENTED_EDGE('',*,*,#3117,.F.);
#4334=ORIENTED_EDGE('',*,*,#3121,.T.);
#4335=ORIENTED_EDGE('',*,*,#3070,.F.);
#4336=ORIENTED_EDGE('',*,*,#2658,.F.);
#4337=ORIENTED_EDGE('',*,*,#3066,.F.);
#4338=ORIENTED_EDGE('',*,*,#3068,.F.);
#4339=ORIENTED_EDGE('',*,*,#3091,.F.);
#4340=ORIENTED_EDGE('',*,*,#3083,.F.);
#4341=ORIENTED_EDGE('',*,*,#3088,.F.);
#4342=ORIENTED_EDGE('',*,*,#2681,.F.);
#4343=ORIENTED_EDGE('',*,*,#3120,.F.);
#4344=ORIENTED_EDGE('',*,*,#2662,.F.);
#4345=ORIENTED_EDGE('',*,*,#3116,.F.);
#4346=ORIENTED_EDGE('',*,*,#3118,.F.);
#4347=ORIENTED_EDGE('',*,*,#3050,.F.);
#4348=ORIENTED_EDGE('',*,*,#2678,.F.);
#4349=ORIENTED_EDGE('',*,*,#3046,.F.);
#4350=ORIENTED_EDGE('',*,*,#3048,.F.);
#4351=ORIENTED_EDGE('',*,*,#3111,.F.);
#4352=ORIENTED_EDGE('',*,*,#3103,.F.);
#4353=ORIENTED_EDGE('',*,*,#3108,.F.);
#4354=ORIENTED_EDGE('',*,*,#2665,.F.);
#4355=ORIENTED_EDGE('',*,*,#3101,.F.);
#4356=ORIENTED_EDGE('',*,*,#3093,.F.);
#4357=ORIENTED_EDGE('',*,*,#3098,.F.);
#4358=ORIENTED_EDGE('',*,*,#2673,.F.);
#4359=ORIENTED_EDGE('',*,*,#3081,.F.);
#4360=ORIENTED_EDGE('',*,*,#3073,.F.);
#4361=ORIENTED_EDGE('',*,*,#3078,.F.);
#4362=ORIENTED_EDGE('',*,*,#2669,.F.);
#4363=ORIENTED_EDGE('',*,*,#3061,.F.);
#4364=ORIENTED_EDGE('',*,*,#3053,.F.);
#4365=ORIENTED_EDGE('',*,*,#3058,.F.);
#4366=ORIENTED_EDGE('',*,*,#2685,.F.);
#4367=ORIENTED_EDGE('',*,*,#3114,.F.);
#4368=ORIENTED_EDGE('',*,*,#3011,.F.);
#4369=ORIENTED_EDGE('',*,*,#3121,.F.);
#4370=ORIENTED_EDGE('',*,*,#3119,.F.);
#4371=ORIENTED_EDGE('',*,*,#3106,.F.);
#4372=ORIENTED_EDGE('',*,*,#3105,.F.);
#4373=ORIENTED_EDGE('',*,*,#3110,.F.);
#4374=ORIENTED_EDGE('',*,*,#3014,.F.);
#4375=ORIENTED_EDGE('',*,*,#3096,.F.);
#4376=ORIENTED_EDGE('',*,*,#3095,.F.);
#4377=ORIENTED_EDGE('',*,*,#3100,.F.);
#4378=ORIENTED_EDGE('',*,*,#3018,.F.);
#4379=ORIENTED_EDGE('',*,*,#3086,.F.);
#4380=ORIENTED_EDGE('',*,*,#3085,.F.);
#4381=ORIENTED_EDGE('',*,*,#3090,.F.);
#4382=ORIENTED_EDGE('',*,*,#3022,.F.);
#4383=ORIENTED_EDGE('',*,*,#3076,.F.);
#4384=ORIENTED_EDGE('',*,*,#3075,.F.);
#4385=ORIENTED_EDGE('',*,*,#3080,.F.);
#4386=ORIENTED_EDGE('',*,*,#3026,.F.);
#4387=ORIENTED_EDGE('',*,*,#3064,.F.);
#4388=ORIENTED_EDGE('',*,*,#3031,.F.);
#4389=ORIENTED_EDGE('',*,*,#3071,.F.);
#4390=ORIENTED_EDGE('',*,*,#3069,.F.);
#4391=ORIENTED_EDGE('',*,*,#3056,.F.);
#4392=ORIENTED_EDGE('',*,*,#3055,.F.);
#4393=ORIENTED_EDGE('',*,*,#3060,.F.);
#4394=ORIENTED_EDGE('',*,*,#3034,.F.);
#4395=ORIENTED_EDGE('',*,*,#3044,.F.);
#4396=ORIENTED_EDGE('',*,*,#3039,.F.);
#4397=ORIENTED_EDGE('',*,*,#3051,.F.);
#4398=ORIENTED_EDGE('',*,*,#3049,.F.);
#4399=ORIENTED_EDGE('',*,*,#2833,.F.);
#4400=ORIENTED_EDGE('',*,*,#2822,.F.);
#4401=ORIENTED_EDGE('',*,*,#2849,.F.);
#4402=ORIENTED_EDGE('',*,*,#2862,.F.);
#4719=PLANE('',#5309);
#4720=PLANE('',#5310);
#4721=PLANE('',#5311);
#4722=PLANE('',#5312);
#4723=PLANE('',#5313);
#4724=PLANE('',#5314);
#4725=PLANE('',#5315);
#4726=PLANE('',#5316);
#4727=PLANE('',#5317);
#4728=PLANE('',#5318);
#4729=PLANE('',#5319);
#4730=PLANE('',#5321);
#4731=PLANE('',#5323);
#4732=PLANE('',#5325);
#4733=PLANE('',#5327);
#4734=PLANE('',#5329);
#4735=PLANE('',#5331);
#4736=PLANE('',#5332);
#4737=PLANE('',#5334);
#4738=PLANE('',#5336);
#4739=PLANE('',#5338);
#4740=PLANE('',#5339);
#4741=PLANE('',#5340);
#4742=PLANE('',#5341);
#4743=PLANE('',#5343);
#4744=PLANE('',#5345);
#4745=PLANE('',#5347);
#4746=PLANE('',#5348);
#4747=PLANE('',#5349);
#4748=PLANE('',#5350);
#4749=PLANE('',#5352);
#4750=PLANE('',#5354);
#4751=PLANE('',#5355);
#4752=PLANE('',#5356);
#4753=PLANE('',#5357);
#4754=PLANE('',#5358);
#4755=PLANE('',#5359);
#4756=PLANE('',#5360);
#4757=PLANE('',#5361);
#4758=PLANE('',#5365);
#4759=PLANE('',#5371);
#4760=PLANE('',#5375);
#4761=PLANE('',#5381);
#4762=PLANE('',#5382);
#4763=PLANE('',#5383);
#4764=PLANE('',#5389);
#4765=PLANE('',#5390);
#4766=PLANE('',#5392);
#4767=PLANE('',#5394);
#4768=PLANE('',#5396);
#4769=PLANE('',#5398);
#4770=PLANE('',#5400);
#4771=PLANE('',#5402);
#4772=PLANE('',#5403);
#4773=PLANE('',#5405);
#4774=PLANE('',#5407);
#4775=PLANE('',#5409);
#4776=PLANE('',#5411);
#4777=PLANE('',#5413);
#4778=PLANE('',#5431);
#4779=PLANE('',#5434);
#4780=PLANE('',#5435);
#4781=PLANE('',#5438);
#4782=PLANE('',#5439);
#4783=PLANE('',#5442);
#4784=PLANE('',#5445);
#4785=PLANE('',#5448);
#4786=PLANE('',#5449);
#4787=PLANE('',#5452);
#4788=PLANE('',#5455);
#4789=PLANE('',#5456);
#4790=PLANE('',#5459);
#4791=PLANE('',#5462);
#4792=PLANE('',#5463);
#4793=PLANE('',#5466);
#4794=PLANE('',#5469);
#4795=PLANE('',#5470);
#4796=PLANE('',#5473);
#4797=PLANE('',#5474);
#4798=PLANE('',#5477);
#4799=PLANE('',#5480);
#4800=PLANE('',#5481);
#4801=PLANE('',#5484);
#4802=PLANE('',#5503);
#4803=PLANE('',#5505);
#4804=PLANE('',#5506);
#4805=PLANE('',#5508);
#4806=PLANE('',#5509);
#4807=PLANE('',#5511);
#4808=PLANE('',#5513);
#4809=PLANE('',#5515);
#4810=PLANE('',#5516);
#4811=PLANE('',#5518);
#4812=PLANE('',#5519);
#4813=PLANE('',#5521);
#4814=PLANE('',#5522);
#4815=PLANE('',#5523);
#4816=PLANE('',#5524);
#4817=PLANE('',#5542);
#4818=PLANE('',#5543);
#4819=PLANE('',#5546);
#4820=PLANE('',#5547);
#4821=PLANE('',#5550);
#4822=PLANE('',#5551);
#4823=PLANE('',#5554);
#4824=PLANE('',#5555);
#4825=PLANE('',#5558);
#4826=PLANE('',#5559);
#4827=PLANE('',#5562);
#4828=PLANE('',#5563);
#4829=PLANE('',#5566);
#4830=PLANE('',#5567);
#4831=PLANE('',#5570);
#4832=PLANE('',#5571);
#4833=PLANE('',#5574);
#4834=PLANE('',#5575);
#4835=PLANE('',#5578);
#4836=PLANE('',#5579);
#4837=PLANE('',#5582);
#4838=PLANE('',#5583);
#4839=PLANE('',#5586);
#4840=PLANE('',#5587);
#4841=PLANE('',#5590);
#4842=PLANE('',#5591);
#4843=PLANE('',#5594);
#4844=PLANE('',#5595);
#4845=PLANE('',#5598);
#4846=PLANE('',#5599);
#4847=PLANE('',#5602);
#4848=PLANE('',#5603);
#4903=ADVANCED_FACE('',(#330),#4719,.F.);
#4904=ADVANCED_FACE('',(#331),#4720,.F.);
#4905=ADVANCED_FACE('',(#332),#4721,.F.);
#4906=ADVANCED_FACE('',(#333),#4722,.T.);
#4907=ADVANCED_FACE('',(#334),#4723,.T.);
#4908=ADVANCED_FACE('',(#335),#4724,.T.);
#4909=ADVANCED_FACE('',(#336),#4725,.T.);
#4910=ADVANCED_FACE('',(#337),#4726,.T.);
#4911=ADVANCED_FACE('',(#338),#4727,.T.);
#4912=ADVANCED_FACE('',(#339,#242,#243,#244,#245,#246,#247,#248,#249),#4728,
 .F.);
#4913=ADVANCED_FACE('',(#340),#4729,.T.);
#4914=ADVANCED_FACE('',(#341),#4730,.F.);
#4915=ADVANCED_FACE('',(#342),#4731,.T.);
#4916=ADVANCED_FACE('',(#343),#4732,.F.);
#4917=ADVANCED_FACE('',(#344),#4733,.T.);
#4918=ADVANCED_FACE('',(#345),#4734,.T.);
#4919=ADVANCED_FACE('',(#346),#4735,.F.);
#4920=ADVANCED_FACE('',(#347),#4736,.F.);
#4921=ADVANCED_FACE('',(#348),#4737,.T.);
#4922=ADVANCED_FACE('',(#349),#4738,.F.);
#4923=ADVANCED_FACE('',(#350),#4739,.T.);
#4924=ADVANCED_FACE('',(#351),#4740,.T.);
#4925=ADVANCED_FACE('',(#352,#250,#251,#252,#253,#254,#255,#256,#257),#4741,
 .T.);
#4926=ADVANCED_FACE('',(#353),#4742,.T.);
#4927=ADVANCED_FACE('',(#354),#4743,.F.);
#4928=ADVANCED_FACE('',(#355),#4744,.F.);
#4929=ADVANCED_FACE('',(#356),#4745,.F.);
#4930=ADVANCED_FACE('',(#357),#4746,.F.);
#4931=ADVANCED_FACE('',(#358),#4747,.F.);
#4932=ADVANCED_FACE('',(#359),#4748,.T.);
#4933=ADVANCED_FACE('',(#360),#4749,.F.);
#4934=ADVANCED_FACE('',(#361),#4750,.F.);
#4935=ADVANCED_FACE('',(#362),#4751,.T.);
#4936=ADVANCED_FACE('',(#363),#4752,.T.);
#4937=ADVANCED_FACE('',(#364),#4753,.T.);
#4938=ADVANCED_FACE('',(#365),#4754,.T.);
#4939=ADVANCED_FACE('',(#366),#4755,.F.);
#4940=ADVANCED_FACE('',(#367),#4756,.T.);
#4941=ADVANCED_FACE('',(#368),#4757,.F.);
#4942=ADVANCED_FACE('',(#369,#258,#259,#260,#261,#262),#4758,.F.);
#4943=ADVANCED_FACE('',(#370),#4759,.T.);
#4944=ADVANCED_FACE('',(#371,#263,#264,#265,#266,#267),#4760,.T.);
#4945=ADVANCED_FACE('',(#372),#4761,.T.);
#4946=ADVANCED_FACE('',(#373),#4762,.F.);
#4947=ADVANCED_FACE('',(#374),#4763,.F.);
#4948=ADVANCED_FACE('',(#375),#165,.F.);
#4949=ADVANCED_FACE('',(#376),#166,.F.);
#4950=ADVANCED_FACE('',(#377),#167,.F.);
#4951=ADVANCED_FACE('',(#378),#168,.F.);
#4952=ADVANCED_FACE('',(#379),#169,.F.);
#4953=ADVANCED_FACE('',(#380),#4764,.F.);
#4954=ADVANCED_FACE('',(#381),#4765,.T.);
#4955=ADVANCED_FACE('',(#382),#4766,.T.);
#4956=ADVANCED_FACE('',(#383),#4767,.F.);
#4957=ADVANCED_FACE('',(#384),#4768,.T.);
#4958=ADVANCED_FACE('',(#385),#4769,.F.);
#4959=ADVANCED_FACE('',(#386),#4770,.T.);
#4960=ADVANCED_FACE('',(#387),#4771,.F.);
#4961=ADVANCED_FACE('',(#388),#4772,.F.);
#4962=ADVANCED_FACE('',(#389),#4773,.T.);
#4963=ADVANCED_FACE('',(#390),#4774,.F.);
#4964=ADVANCED_FACE('',(#391),#4775,.T.);
#4965=ADVANCED_FACE('',(#392),#4776,.F.);
#4966=ADVANCED_FACE('',(#393),#4777,.T.);
#4967=ADVANCED_FACE('',(#394,#268,#269,#270,#271,#272,#273,#274,#275),#170,
 .F.);
#4968=ADVANCED_FACE('',(#395),#4778,.F.);
#4969=ADVANCED_FACE('',(#396),#4779,.F.);
#4970=ADVANCED_FACE('',(#397),#4780,.T.);
#4971=ADVANCED_FACE('',(#398),#4781,.T.);
#4972=ADVANCED_FACE('',(#399),#4782,.F.);
#4973=ADVANCED_FACE('',(#400),#4783,.T.);
#4974=ADVANCED_FACE('',(#401),#4784,.F.);
#4975=ADVANCED_FACE('',(#402),#4785,.F.);
#4976=ADVANCED_FACE('',(#403),#4786,.T.);
#4977=ADVANCED_FACE('',(#404),#4787,.F.);
#4978=ADVANCED_FACE('',(#405),#4788,.F.);
#4979=ADVANCED_FACE('',(#406),#4789,.T.);
#4980=ADVANCED_FACE('',(#407),#4790,.F.);
#4981=ADVANCED_FACE('',(#408),#4791,.F.);
#4982=ADVANCED_FACE('',(#409),#4792,.T.);
#4983=ADVANCED_FACE('',(#410),#4793,.F.);
#4984=ADVANCED_FACE('',(#411),#4794,.F.);
#4985=ADVANCED_FACE('',(#412),#4795,.T.);
#4986=ADVANCED_FACE('',(#413),#4796,.T.);
#4987=ADVANCED_FACE('',(#414),#4797,.F.);
#4988=ADVANCED_FACE('',(#415),#4798,.T.);
#4989=ADVANCED_FACE('',(#416),#4799,.T.);
#4990=ADVANCED_FACE('',(#417),#4800,.F.);
#4991=ADVANCED_FACE('',(#418),#4801,.T.);
#4992=ADVANCED_FACE('',(#419),#171,.T.);
#4993=ADVANCED_FACE('',(#420),#172,.T.);
#4994=ADVANCED_FACE('',(#421),#173,.T.);
#4995=ADVANCED_FACE('',(#422),#174,.T.);
#4996=ADVANCED_FACE('',(#423),#175,.T.);
#4997=ADVANCED_FACE('',(#424),#176,.T.);
#4998=ADVANCED_FACE('',(#425),#177,.T.);
#4999=ADVANCED_FACE('',(#426),#178,.T.);
#5000=ADVANCED_FACE('',(#427),#179,.T.);
#5001=ADVANCED_FACE('',(#428),#180,.T.);
#5002=ADVANCED_FACE('',(#429),#181,.T.);
#5003=ADVANCED_FACE('',(#430),#182,.T.);
#5004=ADVANCED_FACE('',(#431),#183,.T.);
#5005=ADVANCED_FACE('',(#432),#184,.T.);
#5006=ADVANCED_FACE('',(#433),#185,.T.);
#5007=ADVANCED_FACE('',(#434),#186,.T.);
#5008=ADVANCED_FACE('',(#435),#4802,.T.);
#5009=ADVANCED_FACE('',(#436),#4803,.F.);
#5010=ADVANCED_FACE('',(#437),#4804,.F.);
#5011=ADVANCED_FACE('',(#438),#4805,.F.);
#5012=ADVANCED_FACE('',(#439),#4806,.F.);
#5013=ADVANCED_FACE('',(#440),#4807,.F.);
#5014=ADVANCED_FACE('',(#441),#4808,.T.);
#5015=ADVANCED_FACE('',(#442),#4809,.F.);
#5016=ADVANCED_FACE('',(#443),#4810,.T.);
#5017=ADVANCED_FACE('',(#444),#4811,.F.);
#5018=ADVANCED_FACE('',(#445),#4812,.F.);
#5019=ADVANCED_FACE('',(#446),#4813,.T.);
#5020=ADVANCED_FACE('',(#447),#4814,.T.);
#5021=ADVANCED_FACE('',(#448),#4815,.T.);
#5022=ADVANCED_FACE('',(#449),#4816,.T.);
#5023=ADVANCED_FACE('',(#450,#276,#277,#278,#279,#280,#281,#282,#283),#187,
 .F.);
#5024=ADVANCED_FACE('',(#451),#4817,.T.);
#5025=ADVANCED_FACE('',(#452),#4818,.F.);
#5026=ADVANCED_FACE('',(#453),#4819,.F.);
#5027=ADVANCED_FACE('',(#454),#4820,.T.);
#5028=ADVANCED_FACE('',(#455),#4821,.T.);
#5029=ADVANCED_FACE('',(#456),#4822,.F.);
#5030=ADVANCED_FACE('',(#457),#4823,.F.);
#5031=ADVANCED_FACE('',(#458),#4824,.T.);
#5032=ADVANCED_FACE('',(#459),#4825,.T.);
#5033=ADVANCED_FACE('',(#460),#4826,.F.);
#5034=ADVANCED_FACE('',(#461),#4827,.F.);
#5035=ADVANCED_FACE('',(#462),#4828,.T.);
#5036=ADVANCED_FACE('',(#463),#4829,.T.);
#5037=ADVANCED_FACE('',(#464),#4830,.F.);
#5038=ADVANCED_FACE('',(#465),#4831,.F.);
#5039=ADVANCED_FACE('',(#466),#4832,.T.);
#5040=ADVANCED_FACE('',(#467),#4833,.T.);
#5041=ADVANCED_FACE('',(#468),#4834,.F.);
#5042=ADVANCED_FACE('',(#469),#4835,.F.);
#5043=ADVANCED_FACE('',(#470),#4836,.T.);
#5044=ADVANCED_FACE('',(#471),#4837,.T.);
#5045=ADVANCED_FACE('',(#472),#4838,.F.);
#5046=ADVANCED_FACE('',(#473),#4839,.F.);
#5047=ADVANCED_FACE('',(#474),#4840,.T.);
#5048=ADVANCED_FACE('',(#475),#4841,.T.);
#5049=ADVANCED_FACE('',(#476),#4842,.F.);
#5050=ADVANCED_FACE('',(#477),#4843,.F.);
#5051=ADVANCED_FACE('',(#478),#4844,.T.);
#5052=ADVANCED_FACE('',(#479),#4845,.T.);
#5053=ADVANCED_FACE('',(#480),#4846,.F.);
#5054=ADVANCED_FACE('',(#481),#4847,.F.);
#5055=ADVANCED_FACE('',(#482),#4848,.T.);
#5056=ADVANCED_FACE('',(#483),#188,.T.);
#5057=ADVANCED_FACE('',(#484),#189,.T.);
#5058=ADVANCED_FACE('',(#485),#190,.T.);
#5059=ADVANCED_FACE('',(#486),#191,.T.);
#5060=ADVANCED_FACE('',(#487),#192,.T.);
#5061=ADVANCED_FACE('',(#488),#193,.T.);
#5062=ADVANCED_FACE('',(#489),#194,.T.);
#5063=ADVANCED_FACE('',(#490),#195,.T.);
#5064=ADVANCED_FACE('',(#491),#196,.T.);
#5065=ADVANCED_FACE('',(#492),#197,.T.);
#5066=ADVANCED_FACE('',(#493),#198,.T.);
#5067=ADVANCED_FACE('',(#494),#199,.T.);
#5068=ADVANCED_FACE('',(#495),#200,.T.);
#5069=ADVANCED_FACE('',(#496),#201,.T.);
#5070=ADVANCED_FACE('',(#497),#202,.T.);
#5071=ADVANCED_FACE('',(#498),#203,.T.);
#5072=ADVANCED_FACE('',(#499),#204,.F.);
#5151=CLOSED_SHELL('',(#4903,#4904,#4905,#4906,#4907,#4908,#4909,#4910,
#4911,#4912,#4913,#4914,#4915,#4916,#4917,#4918,#4919,#4920,#4921,#4922,
#4923,#4924,#4925,#4926,#4927,#4928,#4929,#4930,#4931,#4932,#4933,#4934,
#4935,#4936,#4937,#4938,#4939,#4940,#4941,#4942,#4943,#4944,#4945,#4946,
#4947,#4948,#4949,#4950,#4951,#4952,#4953,#4954,#4955,#4956,#4957,#4958,
#4959,#4960,#4961,#4962,#4963,#4964,#4965,#4966,#4967,#4968,#4969,#4970,
#4971,#4972,#4973,#4974,#4975,#4976,#4977,#4978,#4979,#4980,#4981,#4982,
#4983,#4984,#4985,#4986,#4987,#4988,#4989,#4990,#4991,#4992,#4993,#4994,
#4995,#4996,#4997,#4998,#4999,#5000,#5001,#5002,#5003,#5004,#5005,#5006,
#5007,#5008,#5009,#5010,#5011,#5012,#5013,#5014,#5015,#5016,#5017,#5018,
#5019,#5020,#5021,#5022,#5023,#5024,#5025,#5026,#5027,#5028,#5029,#5030,
#5031,#5032,#5033,#5034,#5035,#5036,#5037,#5038,#5039,#5040,#5041,#5042,
#5043,#5044,#5045,#5046,#5047,#5048,#5049,#5050,#5051,#5052,#5053,#5054,
#5055,#5056,#5057,#5058,#5059,#5060,#5061,#5062,#5063,#5064,#5065,#5066,
#5067,#5068,#5069,#5070,#5071,#5072));
#5308=AXIS2_PLACEMENT_3D('',#7531,#5947,#5948);
#5309=AXIS2_PLACEMENT_3D('',#7532,#5949,#5950);
#5310=AXIS2_PLACEMENT_3D('',#7541,#5955,#5956);
#5311=AXIS2_PLACEMENT_3D('',#7550,#5961,#5962);
#5312=AXIS2_PLACEMENT_3D('',#7553,#5965,#5966);
#5313=AXIS2_PLACEMENT_3D('',#7567,#5974,#5975);
#5314=AXIS2_PLACEMENT_3D('',#7581,#5983,#5984);
#5315=AXIS2_PLACEMENT_3D('',#7587,#5988,#5989);
#5316=AXIS2_PLACEMENT_3D('',#7596,#5994,#5995);
#5317=AXIS2_PLACEMENT_3D('',#7602,#5999,#6000);
#5318=AXIS2_PLACEMENT_3D('',#7608,#6004,#6005);
#5319=AXIS2_PLACEMENT_3D('',#7676,#6040,#6041);
#5320=AXIS2_PLACEMENT_3D('',#7679,#6042,#6043);
#5321=AXIS2_PLACEMENT_3D('',#7683,#6046,#6047);
#5322=AXIS2_PLACEMENT_3D('',#7688,#6049,#6050);
#5323=AXIS2_PLACEMENT_3D('',#7690,#6052,#6053);
#5324=AXIS2_PLACEMENT_3D('',#7693,#6054,#6055);
#5325=AXIS2_PLACEMENT_3D('',#7697,#6058,#6059);
#5326=AXIS2_PLACEMENT_3D('',#7702,#6061,#6062);
#5327=AXIS2_PLACEMENT_3D('',#7704,#6064,#6065);
#5328=AXIS2_PLACEMENT_3D('',#7707,#6066,#6067);
#5329=AXIS2_PLACEMENT_3D('',#7711,#6070,#6071);
#5330=AXIS2_PLACEMENT_3D('',#7714,#6072,#6073);
#5331=AXIS2_PLACEMENT_3D('',#7718,#6076,#6077);
#5332=AXIS2_PLACEMENT_3D('',#7724,#6081,#6082);
#5333=AXIS2_PLACEMENT_3D('',#7729,#6084,#6085);
#5334=AXIS2_PLACEMENT_3D('',#7731,#6087,#6088);
#5335=AXIS2_PLACEMENT_3D('',#7734,#6089,#6090);
#5336=AXIS2_PLACEMENT_3D('',#7738,#6093,#6094);
#5337=AXIS2_PLACEMENT_3D('',#7743,#6096,#6097);
#5338=AXIS2_PLACEMENT_3D('',#7745,#6099,#6100);
#5339=AXIS2_PLACEMENT_3D('',#7763,#6113,#6114);
#5340=AXIS2_PLACEMENT_3D('',#7766,#6117,#6118);
#5341=AXIS2_PLACEMENT_3D('',#7834,#6153,#6154);
#5342=AXIS2_PLACEMENT_3D('',#7837,#6155,#6156);
#5343=AXIS2_PLACEMENT_3D('',#7841,#6159,#6160);
#5344=AXIS2_PLACEMENT_3D('',#7846,#6162,#6163);
#5345=AXIS2_PLACEMENT_3D('',#7848,#6165,#6166);
#5346=AXIS2_PLACEMENT_3D('',#7853,#6168,#6169);
#5347=AXIS2_PLACEMENT_3D('',#7855,#6171,#6172);
#5348=AXIS2_PLACEMENT_3D('',#7864,#6177,#6178);
#5349=AXIS2_PLACEMENT_3D('',#7873,#6183,#6184);
#5350=AXIS2_PLACEMENT_3D('',#7882,#6189,#6190);
#5351=AXIS2_PLACEMENT_3D('',#7885,#6191,#6192);
#5352=AXIS2_PLACEMENT_3D('',#7889,#6195,#6196);
#5353=AXIS2_PLACEMENT_3D('',#7894,#6198,#6199);
#5354=AXIS2_PLACEMENT_3D('',#7896,#6201,#6202);
#5355=AXIS2_PLACEMENT_3D('',#7905,#6207,#6208);
#5356=AXIS2_PLACEMENT_3D('',#7908,#6211,#6212);
#5357=AXIS2_PLACEMENT_3D('',#7914,#6216,#6217);
#5358=AXIS2_PLACEMENT_3D('',#7917,#6220,#6221);
#5359=AXIS2_PLACEMENT_3D('',#7946,#6238,#6239);
#5360=AXIS2_PLACEMENT_3D('',#7952,#6243,#6244);
#5361=AXIS2_PLACEMENT_3D('',#7959,#6249,#6250);
#5362=AXIS2_PLACEMENT_3D('',#7961,#6251,#6252);
#5363=AXIS2_PLACEMENT_3D('',#7969,#6257,#6258);
#5364=AXIS2_PLACEMENT_3D('',#7974,#6261,#6262);
#5365=AXIS2_PLACEMENT_3D('',#7976,#6264,#6265);
#5366=AXIS2_PLACEMENT_3D('',#7979,#6267,#6268);
#5367=AXIS2_PLACEMENT_3D('',#7981,#6269,#6270);
#5368=AXIS2_PLACEMENT_3D('',#7983,#6271,#6272);
#5369=AXIS2_PLACEMENT_3D('',#7985,#6273,#6274);
#5370=AXIS2_PLACEMENT_3D('',#7987,#6275,#6276);
#5371=AXIS2_PLACEMENT_3D('',#7988,#6277,#6278);
#5372=AXIS2_PLACEMENT_3D('',#7991,#6280,#6281);
#5373=AXIS2_PLACEMENT_3D('',#7993,#6282,#6283);
#5374=AXIS2_PLACEMENT_3D('',#7998,#6286,#6287);
#5375=AXIS2_PLACEMENT_3D('',#7999,#6288,#6289);
#5376=AXIS2_PLACEMENT_3D('',#8001,#6290,#6291);
#5377=AXIS2_PLACEMENT_3D('',#8003,#6292,#6293);
#5378=AXIS2_PLACEMENT_3D('',#8005,#6294,#6295);
#5379=AXIS2_PLACEMENT_3D('',#8007,#6296,#6297);
#5380=AXIS2_PLACEMENT_3D('',#8009,#6298,#6299);
#5381=AXIS2_PLACEMENT_3D('',#8010,#6300,#6301);
#5382=AXIS2_PLACEMENT_3D('',#8012,#6303,#6304);
#5383=AXIS2_PLACEMENT_3D('',#8014,#6306,#6307);
#5384=AXIS2_PLACEMENT_3D('',#8015,#6308,#6309);
#5385=AXIS2_PLACEMENT_3D('',#8017,#6311,#6312);
#5386=AXIS2_PLACEMENT_3D('',#8019,#6314,#6315);
#5387=AXIS2_PLACEMENT_3D('',#8021,#6317,#6318);
#5388=AXIS2_PLACEMENT_3D('',#8023,#6320,#6321);
#5389=AXIS2_PLACEMENT_3D('',#8025,#6323,#6324);
#5390=AXIS2_PLACEMENT_3D('',#8028,#6327,#6328);
#5391=AXIS2_PLACEMENT_3D('',#8030,#6329,#6330);
#5392=AXIS2_PLACEMENT_3D('',#8032,#6332,#6333);
#5393=AXIS2_PLACEMENT_3D('',#8033,#6334,#6335);
#5394=AXIS2_PLACEMENT_3D('',#8034,#6336,#6337);
#5395=AXIS2_PLACEMENT_3D('',#8035,#6338,#6339);
#5396=AXIS2_PLACEMENT_3D('',#8036,#6340,#6341);
#5397=AXIS2_PLACEMENT_3D('',#8037,#6342,#6343);
#5398=AXIS2_PLACEMENT_3D('',#8038,#6344,#6345);
#5399=AXIS2_PLACEMENT_3D('',#8039,#6346,#6347);
#5400=AXIS2_PLACEMENT_3D('',#8040,#6348,#6349);
#5401=AXIS2_PLACEMENT_3D('',#8043,#6350,#6351);
#5402=AXIS2_PLACEMENT_3D('',#8047,#6354,#6355);
#5403=AXIS2_PLACEMENT_3D('',#8053,#6359,#6360);
#5404=AXIS2_PLACEMENT_3D('',#8055,#6361,#6362);
#5405=AXIS2_PLACEMENT_3D('',#8057,#6364,#6365);
#5406=AXIS2_PLACEMENT_3D('',#8058,#6366,#6367);
#5407=AXIS2_PLACEMENT_3D('',#8059,#6368,#6369);
#5408=AXIS2_PLACEMENT_3D('',#8060,#6370,#6371);
#5409=AXIS2_PLACEMENT_3D('',#8061,#6372,#6373);
#5410=AXIS2_PLACEMENT_3D('',#8062,#6374,#6375);
#5411=AXIS2_PLACEMENT_3D('',#8063,#6376,#6377);
#5412=AXIS2_PLACEMENT_3D('',#8064,#6378,#6379);
#5413=AXIS2_PLACEMENT_3D('',#8065,#6380,#6381);
#5414=AXIS2_PLACEMENT_3D('',#8071,#6387,#6388);
#5415=AXIS2_PLACEMENT_3D('',#8074,#6389,#6390);
#5416=AXIS2_PLACEMENT_3D('',#8078,#6392,#6393);
#5417=AXIS2_PLACEMENT_3D('',#8082,#6395,#6396);
#5418=AXIS2_PLACEMENT_3D('',#8086,#6398,#6399);
#5419=AXIS2_PLACEMENT_3D('',#8092,#6402,#6403);
#5420=AXIS2_PLACEMENT_3D('',#8095,#6405,#6406);
#5421=AXIS2_PLACEMENT_3D('',#8100,#6408,#6409);
#5422=AXIS2_PLACEMENT_3D('',#8103,#6411,#6412);
#5423=AXIS2_PLACEMENT_3D('',#8108,#6414,#6415);
#5424=AXIS2_PLACEMENT_3D('',#8111,#6417,#6418);
#5425=AXIS2_PLACEMENT_3D('',#8116,#6420,#6421);
#5426=AXIS2_PLACEMENT_3D('',#8119,#6423,#6424);
#5427=AXIS2_PLACEMENT_3D('',#8122,#6425,#6426);
#5428=AXIS2_PLACEMENT_3D('',#8126,#6428,#6429);
#5429=AXIS2_PLACEMENT_3D('',#8132,#6432,#6433);
#5430=AXIS2_PLACEMENT_3D('',#8135,#6435,#6436);
#5431=AXIS2_PLACEMENT_3D('',#8136,#6437,#6438);
#5432=AXIS2_PLACEMENT_3D('',#8138,#6439,#6440);
#5433=AXIS2_PLACEMENT_3D('',#8139,#6441,#6442);
#5434=AXIS2_PLACEMENT_3D('',#8141,#6444,#6445);
#5435=AXIS2_PLACEMENT_3D('',#8143,#6447,#6448);
#5436=AXIS2_PLACEMENT_3D('',#8145,#6449,#6450);
#5437=AXIS2_PLACEMENT_3D('',#8146,#6451,#6452);
#5438=AXIS2_PLACEMENT_3D('',#8147,#6453,#6454);
#5439=AXIS2_PLACEMENT_3D('',#8150,#6457,#6458);
#5440=AXIS2_PLACEMENT_3D('',#8152,#6459,#6460);
#5441=AXIS2_PLACEMENT_3D('',#8153,#6461,#6462);
#5442=AXIS2_PLACEMENT_3D('',#8154,#6463,#6464);
#5443=AXIS2_PLACEMENT_3D('',#8156,#6465,#6466);
#5444=AXIS2_PLACEMENT_3D('',#8157,#6467,#6468);
#5445=AXIS2_PLACEMENT_3D('',#8158,#6469,#6470);
#5446=AXIS2_PLACEMENT_3D('',#8160,#6471,#6472);
#5447=AXIS2_PLACEMENT_3D('',#8161,#6473,#6474);
#5448=AXIS2_PLACEMENT_3D('',#8163,#6476,#6477);
#5449=AXIS2_PLACEMENT_3D('',#8165,#6479,#6480);
#5450=AXIS2_PLACEMENT_3D('',#8167,#6481,#6482);
#5451=AXIS2_PLACEMENT_3D('',#8168,#6483,#6484);
#5452=AXIS2_PLACEMENT_3D('',#8169,#6485,#6486);
#5453=AXIS2_PLACEMENT_3D('',#8171,#6487,#6488);
#5454=AXIS2_PLACEMENT_3D('',#8172,#6489,#6490);
#5455=AXIS2_PLACEMENT_3D('',#8174,#6492,#6493);
#5456=AXIS2_PLACEMENT_3D('',#8176,#6495,#6496);
#5457=AXIS2_PLACEMENT_3D('',#8178,#6497,#6498);
#5458=AXIS2_PLACEMENT_3D('',#8179,#6499,#6500);
#5459=AXIS2_PLACEMENT_3D('',#8180,#6501,#6502);
#5460=AXIS2_PLACEMENT_3D('',#8182,#6503,#6504);
#5461=AXIS2_PLACEMENT_3D('',#8183,#6505,#6506);
#5462=AXIS2_PLACEMENT_3D('',#8185,#6508,#6509);
#5463=AXIS2_PLACEMENT_3D('',#8187,#6511,#6512);
#5464=AXIS2_PLACEMENT_3D('',#8189,#6513,#6514);
#5465=AXIS2_PLACEMENT_3D('',#8190,#6515,#6516);
#5466=AXIS2_PLACEMENT_3D('',#8191,#6517,#6518);
#5467=AXIS2_PLACEMENT_3D('',#8193,#6519,#6520);
#5468=AXIS2_PLACEMENT_3D('',#8194,#6521,#6522);
#5469=AXIS2_PLACEMENT_3D('',#8196,#6524,#6525);
#5470=AXIS2_PLACEMENT_3D('',#8198,#6527,#6528);
#5471=AXIS2_PLACEMENT_3D('',#8200,#6529,#6530);
#5472=AXIS2_PLACEMENT_3D('',#8201,#6531,#6532);
#5473=AXIS2_PLACEMENT_3D('',#8202,#6533,#6534);
#5474=AXIS2_PLACEMENT_3D('',#8205,#6537,#6538);
#5475=AXIS2_PLACEMENT_3D('',#8207,#6539,#6540);
#5476=AXIS2_PLACEMENT_3D('',#8208,#6541,#6542);
#5477=AXIS2_PLACEMENT_3D('',#8209,#6543,#6544);
#5478=AXIS2_PLACEMENT_3D('',#8211,#6545,#6546);
#5479=AXIS2_PLACEMENT_3D('',#8212,#6547,#6548);
#5480=AXIS2_PLACEMENT_3D('',#8213,#6549,#6550);
#5481=AXIS2_PLACEMENT_3D('',#8216,#6553,#6554);
#5482=AXIS2_PLACEMENT_3D('',#8218,#6555,#6556);
#5483=AXIS2_PLACEMENT_3D('',#8219,#6557,#6558);
#5484=AXIS2_PLACEMENT_3D('',#8220,#6559,#6560);
#5485=AXIS2_PLACEMENT_3D('',#8222,#6561,#6562);
#5486=AXIS2_PLACEMENT_3D('',#8223,#6563,#6564);
#5487=AXIS2_PLACEMENT_3D('',#8224,#6565,#6566);
#5488=AXIS2_PLACEMENT_3D('',#8226,#6568,#6569);
#5489=AXIS2_PLACEMENT_3D('',#8227,#6570,#6571);
#5490=AXIS2_PLACEMENT_3D('',#8229,#6573,#6574);
#5491=AXIS2_PLACEMENT_3D('',#8230,#6575,#6576);
#5492=AXIS2_PLACEMENT_3D('',#8232,#6578,#6579);
#5493=AXIS2_PLACEMENT_3D('',#8233,#6580,#6581);
#5494=AXIS2_PLACEMENT_3D('',#8235,#6583,#6584);
#5495=AXIS2_PLACEMENT_3D('',#8236,#6585,#6586);
#5496=AXIS2_PLACEMENT_3D('',#8238,#6588,#6589);
#5497=AXIS2_PLACEMENT_3D('',#8239,#6590,#6591);
#5498=AXIS2_PLACEMENT_3D('',#8241,#6593,#6594);
#5499=AXIS2_PLACEMENT_3D('',#8242,#6595,#6596);
#5500=AXIS2_PLACEMENT_3D('',#8244,#6598,#6599);
#5501=AXIS2_PLACEMENT_3D('',#8245,#6600,#6601);
#5502=AXIS2_PLACEMENT_3D('',#8247,#6603,#6604);
#5503=AXIS2_PLACEMENT_3D('',#8248,#6605,#6606);
#5504=AXIS2_PLACEMENT_3D('',#8251,#6607,#6608);
#5505=AXIS2_PLACEMENT_3D('',#8255,#6611,#6612);
#5506=AXIS2_PLACEMENT_3D('',#8261,#6616,#6617);
#5507=AXIS2_PLACEMENT_3D('',#8263,#6618,#6619);
#5508=AXIS2_PLACEMENT_3D('',#8265,#6621,#6622);
#5509=AXIS2_PLACEMENT_3D('',#8271,#6626,#6627);
#5510=AXIS2_PLACEMENT_3D('',#8273,#6628,#6629);
#5511=AXIS2_PLACEMENT_3D('',#8275,#6631,#6632);
#5512=AXIS2_PLACEMENT_3D('',#8276,#6633,#6634);
#5513=AXIS2_PLACEMENT_3D('',#8277,#6635,#6636);
#5514=AXIS2_PLACEMENT_3D('',#8280,#6637,#6638);
#5515=AXIS2_PLACEMENT_3D('',#8284,#6641,#6642);
#5516=AXIS2_PLACEMENT_3D('',#8287,#6645,#6646);
#5517=AXIS2_PLACEMENT_3D('',#8290,#6647,#6648);
#5518=AXIS2_PLACEMENT_3D('',#8294,#6651,#6652);
#5519=AXIS2_PLACEMENT_3D('',#8300,#6656,#6657);
#5520=AXIS2_PLACEMENT_3D('',#8302,#6658,#6659);
#5521=AXIS2_PLACEMENT_3D('',#8304,#6661,#6662);
#5522=AXIS2_PLACEMENT_3D('',#8306,#6664,#6665);
#5523=AXIS2_PLACEMENT_3D('',#8308,#6667,#6668);
#5524=AXIS2_PLACEMENT_3D('',#8310,#6670,#6671);
#5525=AXIS2_PLACEMENT_3D('',#8316,#6677,#6678);
#5526=AXIS2_PLACEMENT_3D('',#8319,#6679,#6680);
#5527=AXIS2_PLACEMENT_3D('',#8323,#6682,#6683);
#5528=AXIS2_PLACEMENT_3D('',#8329,#6686,#6687);
#5529=AXIS2_PLACEMENT_3D('',#8332,#6689,#6690);
#5530=AXIS2_PLACEMENT_3D('',#8337,#6692,#6693);
#5531=AXIS2_PLACEMENT_3D('',#8340,#6695,#6696);
#5532=AXIS2_PLACEMENT_3D('',#8345,#6698,#6699);
#5533=AXIS2_PLACEMENT_3D('',#8348,#6701,#6702);
#5534=AXIS2_PLACEMENT_3D('',#8353,#6704,#6705);
#5535=AXIS2_PLACEMENT_3D('',#8356,#6707,#6708);
#5536=AXIS2_PLACEMENT_3D('',#8359,#6709,#6710);
#5537=AXIS2_PLACEMENT_3D('',#8363,#6712,#6713);
#5538=AXIS2_PLACEMENT_3D('',#8369,#6716,#6717);
#5539=AXIS2_PLACEMENT_3D('',#8372,#6719,#6720);
#5540=AXIS2_PLACEMENT_3D('',#8375,#6721,#6722);
#5541=AXIS2_PLACEMENT_3D('',#8379,#6724,#6725);
#5542=AXIS2_PLACEMENT_3D('',#8381,#6727,#6728);
#5543=AXIS2_PLACEMENT_3D('',#8384,#6731,#6732);
#5544=AXIS2_PLACEMENT_3D('',#8386,#6733,#6734);
#5545=AXIS2_PLACEMENT_3D('',#8389,#6736,#6737);
#5546=AXIS2_PLACEMENT_3D('',#8390,#6738,#6739);
#5547=AXIS2_PLACEMENT_3D('',#8396,#6743,#6744);
#5548=AXIS2_PLACEMENT_3D('',#8397,#6745,#6746);
#5549=AXIS2_PLACEMENT_3D('',#8398,#6747,#6748);
#5550=AXIS2_PLACEMENT_3D('',#8399,#6749,#6750);
#5551=AXIS2_PLACEMENT_3D('',#8408,#6755,#6756);
#5552=AXIS2_PLACEMENT_3D('',#8409,#6757,#6758);
#5553=AXIS2_PLACEMENT_3D('',#8411,#6760,#6761);
#5554=AXIS2_PLACEMENT_3D('',#8412,#6762,#6763);
#5555=AXIS2_PLACEMENT_3D('',#8414,#6765,#6766);
#5556=AXIS2_PLACEMENT_3D('',#8415,#6767,#6768);
#5557=AXIS2_PLACEMENT_3D('',#8416,#6769,#6770);
#5558=AXIS2_PLACEMENT_3D('',#8417,#6771,#6772);
#5559=AXIS2_PLACEMENT_3D('',#8420,#6775,#6776);
#5560=AXIS2_PLACEMENT_3D('',#8422,#6777,#6778);
#5561=AXIS2_PLACEMENT_3D('',#8425,#6780,#6781);
#5562=AXIS2_PLACEMENT_3D('',#8426,#6782,#6783);
#5563=AXIS2_PLACEMENT_3D('',#8432,#6787,#6788);
#5564=AXIS2_PLACEMENT_3D('',#8433,#6789,#6790);
#5565=AXIS2_PLACEMENT_3D('',#8434,#6791,#6792);
#5566=AXIS2_PLACEMENT_3D('',#8435,#6793,#6794);
#5567=AXIS2_PLACEMENT_3D('',#8444,#6799,#6800);
#5568=AXIS2_PLACEMENT_3D('',#8445,#6801,#6802);
#5569=AXIS2_PLACEMENT_3D('',#8447,#6804,#6805);
#5570=AXIS2_PLACEMENT_3D('',#8448,#6806,#6807);
#5571=AXIS2_PLACEMENT_3D('',#8450,#6809,#6810);
#5572=AXIS2_PLACEMENT_3D('',#8451,#6811,#6812);
#5573=AXIS2_PLACEMENT_3D('',#8452,#6813,#6814);
#5574=AXIS2_PLACEMENT_3D('',#8453,#6815,#6816);
#5575=AXIS2_PLACEMENT_3D('',#8462,#6821,#6822);
#5576=AXIS2_PLACEMENT_3D('',#8463,#6823,#6824);
#5577=AXIS2_PLACEMENT_3D('',#8465,#6826,#6827);
#5578=AXIS2_PLACEMENT_3D('',#8466,#6828,#6829);
#5579=AXIS2_PLACEMENT_3D('',#8468,#6831,#6832);
#5580=AXIS2_PLACEMENT_3D('',#8469,#6833,#6834);
#5581=AXIS2_PLACEMENT_3D('',#8470,#6835,#6836);
#5582=AXIS2_PLACEMENT_3D('',#8471,#6837,#6838);
#5583=AXIS2_PLACEMENT_3D('',#8480,#6843,#6844);
#5584=AXIS2_PLACEMENT_3D('',#8481,#6845,#6846);
#5585=AXIS2_PLACEMENT_3D('',#8483,#6848,#6849);
#5586=AXIS2_PLACEMENT_3D('',#8484,#6850,#6851);
#5587=AXIS2_PLACEMENT_3D('',#8486,#6853,#6854);
#5588=AXIS2_PLACEMENT_3D('',#8487,#6855,#6856);
#5589=AXIS2_PLACEMENT_3D('',#8488,#6857,#6858);
#5590=AXIS2_PLACEMENT_3D('',#8489,#6859,#6860);
#5591=AXIS2_PLACEMENT_3D('',#8498,#6865,#6866);
#5592=AXIS2_PLACEMENT_3D('',#8499,#6867,#6868);
#5593=AXIS2_PLACEMENT_3D('',#8501,#6870,#6871);
#5594=AXIS2_PLACEMENT_3D('',#8502,#6872,#6873);
#5595=AXIS2_PLACEMENT_3D('',#8504,#6875,#6876);
#5596=AXIS2_PLACEMENT_3D('',#8505,#6877,#6878);
#5597=AXIS2_PLACEMENT_3D('',#8506,#6879,#6880);
#5598=AXIS2_PLACEMENT_3D('',#8507,#6881,#6882);
#5599=AXIS2_PLACEMENT_3D('',#8510,#6885,#6886);
#5600=AXIS2_PLACEMENT_3D('',#8512,#6887,#6888);
#5601=AXIS2_PLACEMENT_3D('',#8515,#6890,#6891);
#5602=AXIS2_PLACEMENT_3D('',#8516,#6892,#6893);
#5603=AXIS2_PLACEMENT_3D('',#8522,#6897,#6898);
#5604=AXIS2_PLACEMENT_3D('',#8523,#6899,#6900);
#5605=AXIS2_PLACEMENT_3D('',#8524,#6901,#6902);
#5606=AXIS2_PLACEMENT_3D('',#8525,#6903,#6904);
#5607=AXIS2_PLACEMENT_3D('',#8526,#6905,#6906);
#5608=AXIS2_PLACEMENT_3D('',#8527,#6907,#6908);
#5609=AXIS2_PLACEMENT_3D('',#8528,#6909,#6910);
#5610=AXIS2_PLACEMENT_3D('',#8529,#6911,#6912);
#5611=AXIS2_PLACEMENT_3D('',#8530,#6913,#6914);
#5612=AXIS2_PLACEMENT_3D('',#8531,#6915,#6916);
#5613=AXIS2_PLACEMENT_3D('',#8532,#6917,#6918);
#5614=AXIS2_PLACEMENT_3D('',#8533,#6919,#6920);
#5615=AXIS2_PLACEMENT_3D('',#8534,#6921,#6922);
#5616=AXIS2_PLACEMENT_3D('',#8535,#6923,#6924);
#5617=AXIS2_PLACEMENT_3D('',#8536,#6925,#6926);
#5618=AXIS2_PLACEMENT_3D('',#8537,#6927,#6928);
#5619=AXIS2_PLACEMENT_3D('',#8538,#6929,#6930);
#5620=AXIS2_PLACEMENT_3D('',#8539,#6931,#6932);
#5621=AXIS2_PLACEMENT_3D('',#8540,#6933,#6934);
#5622=AXIS2_PLACEMENT_3D('',#8541,#6935,#6936);
#5947=DIRECTION('axis',(0.,0.,1.));
#5948=DIRECTION('refdir',(1.,0.,0.));
#5949=DIRECTION('center_axis',(-3.49459686471004E-16,-3.44690246421401E-16,
-1.));
#5950=DIRECTION('ref_axis',(-1.34368925898019E-12,-1.,3.44690246421871E-16));
#5951=DIRECTION('',(-3.65204942310907E-16,1.,-3.446902464214E-16));
#5952=DIRECTION('',(-1.,1.34368543743058E-12,3.49459686470541E-16));
#5953=DIRECTION('',(0.,-1.,3.44690246421401E-16));
#5954=DIRECTION('',(1.,0.,-3.49459686471004E-16));
#5955=DIRECTION('center_axis',(3.49459686467822E-16,-2.0237855394456E-15,
1.));
#5956=DIRECTION('ref_axis',(1.34605772573104E-12,1.,2.02378553944513E-15));
#5957=DIRECTION('',(3.65204942310907E-16,-1.,-2.0237855394456E-15));
#5958=DIRECTION('',(-1.,0.,3.49459686467822E-16));
#5959=DIRECTION('',(0.,1.,2.0237855394456E-15));
#5960=DIRECTION('',(-1.,1.34368543743058E-12,3.49459686470541E-16));
#5961=DIRECTION('center_axis',(-1.34368543743058E-12,-1.,-2.02378553944513E-15));
#5962=DIRECTION('ref_axis',(-8.8817159728603E-16,-2.02378553944394E-15,
1.));
#5963=DIRECTION('',(-7.39096481182707E-31,2.02378553944513E-15,-1.));
#5964=DIRECTION('',(0.,-2.02378553944513E-15,1.));
#5965=DIRECTION('center_axis',(0.,1.,0.));
#5966=DIRECTION('ref_axis',(0.,0.,1.));
#5967=DIRECTION('',(0.,0.,-1.));
#5968=DIRECTION('',(1.,0.,0.));
#5969=DIRECTION('',(0.,0.,-1.));
#5970=DIRECTION('',(-1.,0.,0.));
#5971=DIRECTION('',(0.,0.,-1.));
#5972=DIRECTION('',(1.,0.,0.));
#5973=DIRECTION('',(0.,0.,-1.));
#5974=DIRECTION('center_axis',(0.,1.,0.));
#5975=DIRECTION('ref_axis',(0.,0.,1.));
#5976=DIRECTION('',(0.,0.,-1.));
#5977=DIRECTION('',(1.,0.,0.));
#5978=DIRECTION('',(0.,0.,-1.));
#5979=DIRECTION('',(-1.,0.,0.));
#5980=DIRECTION('',(0.,0.,-1.));
#5981=DIRECTION('',(1.,0.,0.));
#5982=DIRECTION('',(0.,0.,-1.));
#5983=DIRECTION('center_axis',(-1.,-3.65204942310907E-16,0.));
#5984=DIRECTION('ref_axis',(3.65204942310907E-16,-1.,0.));
#5985=DIRECTION('',(-3.65204942310907E-16,1.,0.));
#5986=DIRECTION('',(0.,0.,-1.));
#5987=DIRECTION('',(-3.65204942310907E-16,1.,0.));
#5988=DIRECTION('center_axis',(1.34368925898019E-12,1.,-5.08164181815587E-15));
#5989=DIRECTION('ref_axis',(3.55268652758613E-15,-5.08164181816064E-15,
-1.));
#5990=DIRECTION('',(0.,5.08164181815587E-15,1.));
#5991=DIRECTION('',(-1.,1.34368925898019E-12,-2.5823130969E-16));
#5992=DIRECTION('',(-3.55268652758613E-15,5.08164181816065E-15,1.));
#5993=DIRECTION('',(1.,0.,0.));
#5994=DIRECTION('center_axis',(2.5823130969E-16,-3.46795905806759E-28,-1.));
#5995=DIRECTION('ref_axis',(1.,-1.3429252284855E-12,2.5823130969E-16));
#5996=DIRECTION('',(-1.34296614234377E-12,-1.,0.));
#5997=DIRECTION('',(-1.,1.3429252284855E-12,-2.5823130969E-16));
#5998=DIRECTION('',(-1.34296614234377E-12,-1.,0.));
#5999=DIRECTION('center_axis',(1.3429252284855E-12,1.,9.98628687409672E-23));
#6000=DIRECTION('ref_axis',(-1.,1.3429252284855E-12,1.26981758441774E-15));
#6001=DIRECTION('',(1.,-1.34216120476708E-12,2.5823130969E-16));
#6002=DIRECTION('',(-1.26981758441774E-15,9.98645738638139E-23,-1.));
#6003=DIRECTION('',(1.26981758440819E-15,-7.1054274574656E-15,1.));
#6004=DIRECTION('center_axis',(0.,0.,1.));
#6005=DIRECTION('ref_axis',(1.,0.,0.));
#6006=DIRECTION('',(1.82602471155453E-16,-1.,0.));
#6007=DIRECTION('',(1.,0.,0.));
#6008=DIRECTION('',(0.,-1.,0.));
#6009=DIRECTION('',(1.,0.,0.));
#6010=DIRECTION('',(0.,-1.,0.));
#6011=DIRECTION('',(1.,0.,0.));
#6012=DIRECTION('',(0.,-1.,0.));
#6013=DIRECTION('',(1.,5.78241158658936E-16,0.));
#6014=DIRECTION('',(0.,-1.,0.));
#6015=DIRECTION('',(1.,0.,0.));
#6016=DIRECTION('',(1.,0.,0.));
#6017=DIRECTION('',(0.,-1.,0.));
#6018=DIRECTION('',(1.,0.,0.));
#6019=DIRECTION('',(0.,-1.,0.));
#6020=DIRECTION('',(1.,0.,0.));
#6021=DIRECTION('',(1.7347234759768E-16,-1.,0.));
#6022=DIRECTION('',(1.,2.89120579329468E-16,0.));
#6023=DIRECTION('',(0.,-1.,0.));
#6024=DIRECTION('',(1.,0.,0.));
#6025=DIRECTION('',(0.,-1.,0.));
#6026=DIRECTION('',(1.,0.,0.));
#6027=DIRECTION('',(1.7347234759768E-16,-1.,0.));
#6028=DIRECTION('',(0.,-1.,0.));
#6029=DIRECTION('',(1.,0.,0.));
#6030=DIRECTION('',(0.,-1.,0.));
#6031=DIRECTION('',(1.,0.,0.));
#6032=DIRECTION('',(-1.,0.,0.));
#6033=DIRECTION('',(0.,1.,0.));
#6034=DIRECTION('',(-1.,0.,0.));
#6035=DIRECTION('',(-1.7347234759768E-16,1.,0.));
#6036=DIRECTION('',(1.,0.,0.));
#6037=DIRECTION('',(0.,-1.,0.));
#6038=DIRECTION('',(1.,0.,0.));
#6039=DIRECTION('',(0.,-1.,0.));
#6040=DIRECTION('center_axis',(1.,0.,0.));
#6041=DIRECTION('ref_axis',(0.,0.,-1.));
#6042=DIRECTION('center_axis',(1.,0.,0.));
#6043=DIRECTION('ref_axis',(0.,0.,-1.));
#6044=DIRECTION('',(0.,-1.,0.));
#6045=DIRECTION('',(0.,0.,-1.));
#6046=DIRECTION('center_axis',(1.,0.,0.));
#6047=DIRECTION('ref_axis',(0.,0.,-1.));
#6048=DIRECTION('',(0.,-1.,0.));
#6049=DIRECTION('center_axis',(1.,0.,0.));
#6050=DIRECTION('ref_axis',(0.,0.,-1.));
#6051=DIRECTION('',(0.,0.,-1.));
#6052=DIRECTION('center_axis',(1.,0.,0.));
#6053=DIRECTION('ref_axis',(0.,0.,-1.));
#6054=DIRECTION('center_axis',(1.,0.,0.));
#6055=DIRECTION('ref_axis',(0.,0.,-1.));
#6056=DIRECTION('',(0.,-1.,0.));
#6057=DIRECTION('',(0.,0.,-1.));
#6058=DIRECTION('center_axis',(1.,0.,0.));
#6059=DIRECTION('ref_axis',(0.,0.,-1.));
#6060=DIRECTION('',(0.,-1.,0.));
#6061=DIRECTION('center_axis',(1.,0.,0.));
#6062=DIRECTION('ref_axis',(0.,0.,-1.));
#6063=DIRECTION('',(0.,0.,-1.));
#6064=DIRECTION('center_axis',(1.,1.7347234759768E-16,0.));
#6065=DIRECTION('ref_axis',(-1.7347234759768E-16,1.,0.));
#6066=DIRECTION('center_axis',(1.,1.7347234759768E-16,0.));
#6067=DIRECTION('ref_axis',(-1.7347234759768E-16,1.,0.));
#6068=DIRECTION('',(0.,0.,-1.));
#6069=DIRECTION('',(1.7347234759768E-16,-1.,0.));
#6070=DIRECTION('center_axis',(-1.,-1.7347234759768E-16,0.));
#6071=DIRECTION('ref_axis',(1.7347234759768E-16,-1.,0.));
#6072=DIRECTION('center_axis',(-1.,-1.7347234759768E-16,0.));
#6073=DIRECTION('ref_axis',(1.7347234759768E-16,-1.,0.));
#6074=DIRECTION('',(0.,0.,-1.));
#6075=DIRECTION('',(-1.7347234759768E-16,1.,0.));
#6076=DIRECTION('center_axis',(0.,-1.,0.));
#6077=DIRECTION('ref_axis',(0.,0.,-1.));
#6078=DIRECTION('',(-1.,0.,0.));
#6079=DIRECTION('',(0.,0.,-1.));
#6080=DIRECTION('',(-1.,0.,0.));
#6081=DIRECTION('center_axis',(1.,1.7347234759768E-16,0.));
#6082=DIRECTION('ref_axis',(-1.7347234759768E-16,1.,0.));
#6083=DIRECTION('',(0.,0.,-1.));
#6084=DIRECTION('center_axis',(1.,1.7347234759768E-16,0.));
#6085=DIRECTION('ref_axis',(-1.7347234759768E-16,1.,0.));
#6086=DIRECTION('',(1.7347234759768E-16,-1.,0.));
#6087=DIRECTION('center_axis',(1.,0.,0.));
#6088=DIRECTION('ref_axis',(0.,0.,-1.));
#6089=DIRECTION('center_axis',(1.,0.,0.));
#6090=DIRECTION('ref_axis',(0.,0.,-1.));
#6091=DIRECTION('',(0.,-1.,0.));
#6092=DIRECTION('',(0.,0.,-1.));
#6093=DIRECTION('center_axis',(1.,0.,0.));
#6094=DIRECTION('ref_axis',(0.,0.,-1.));
#6095=DIRECTION('',(0.,-1.,0.));
#6096=DIRECTION('center_axis',(1.,0.,0.));
#6097=DIRECTION('ref_axis',(0.,0.,-1.));
#6098=DIRECTION('',(0.,0.,-1.));
#6099=DIRECTION('center_axis',(0.,0.,1.));
#6100=DIRECTION('ref_axis',(1.,0.,0.));
#6101=DIRECTION('',(0.,-1.,0.));
#6102=DIRECTION('',(-1.,0.,0.));
#6103=DIRECTION('',(1.,0.,0.));
#6104=DIRECTION('',(-1.,0.,0.));
#6105=DIRECTION('',(1.,0.,0.));
#6106=DIRECTION('',(-1.,0.,0.));
#6107=DIRECTION('',(0.,1.,0.));
#6108=DIRECTION('',(-1.,0.,0.));
#6109=DIRECTION('',(1.,0.,0.));
#6110=DIRECTION('',(-1.,0.,0.));
#6111=DIRECTION('',(0.,-1.,0.));
#6112=DIRECTION('',(1.,0.,0.));
#6113=DIRECTION('center_axis',(0.,0.,1.));
#6114=DIRECTION('ref_axis',(1.,0.,0.));
#6115=DIRECTION('',(0.,-1.,0.));
#6116=DIRECTION('',(0.,-1.,0.));
#6117=DIRECTION('center_axis',(0.,0.,1.));
#6118=DIRECTION('ref_axis',(1.,0.,0.));
#6119=DIRECTION('',(1.82602471155453E-16,-1.,0.));
#6120=DIRECTION('',(1.,0.,0.));
#6121=DIRECTION('',(0.,-1.,0.));
#6122=DIRECTION('',(-1.,0.,0.));
#6123=DIRECTION('',(0.,-1.,0.));
#6124=DIRECTION('',(-1.,0.,0.));
#6125=DIRECTION('',(-1.,0.,0.));
#6126=DIRECTION('',(0.,-1.,0.));
#6127=DIRECTION('',(-1.,0.,0.));
#6128=DIRECTION('',(0.,-1.,0.));
#6129=DIRECTION('',(1.7347234759768E-16,1.,0.));
#6130=DIRECTION('',(1.,-2.89120579329468E-16,0.));
#6131=DIRECTION('',(0.,1.,0.));
#6132=DIRECTION('',(1.,-1.44560289664734E-16,0.));
#6133=DIRECTION('',(-1.,2.89120579329468E-16,0.));
#6134=DIRECTION('',(-1.7347234759768E-16,-1.,0.));
#6135=DIRECTION('',(-1.,2.89120579329468E-16,0.));
#6136=DIRECTION('',(0.,-1.,0.));
#6137=DIRECTION('',(-1.,0.,0.));
#6138=DIRECTION('',(0.,-1.,0.));
#6139=DIRECTION('',(-1.,0.,0.));
#6140=DIRECTION('',(0.,-1.,0.));
#6141=DIRECTION('',(0.,-1.,0.));
#6142=DIRECTION('',(-1.,0.,0.));
#6143=DIRECTION('',(0.,-1.,0.));
#6144=DIRECTION('',(-1.,0.,0.));
#6145=DIRECTION('',(-1.7347234759768E-16,-1.,0.));
#6146=DIRECTION('',(-1.,0.,0.));
#6147=DIRECTION('',(0.,-1.,0.));
#6148=DIRECTION('',(-1.,0.,0.));
#6149=DIRECTION('',(0.,-1.,0.));
#6150=DIRECTION('',(-1.,5.78241158658936E-16,0.));
#6151=DIRECTION('',(-1.73472347597681E-16,-1.,0.));
#6152=DIRECTION('',(-1.,0.,0.));
#6153=DIRECTION('center_axis',(1.,0.,0.));
#6154=DIRECTION('ref_axis',(0.,0.,-1.));
#6155=DIRECTION('center_axis',(1.,0.,0.));
#6156=DIRECTION('ref_axis',(0.,0.,-1.));
#6157=DIRECTION('',(0.,1.,0.));
#6158=DIRECTION('',(0.,0.,1.));
#6159=DIRECTION('center_axis',(1.,0.,0.));
#6160=DIRECTION('ref_axis',(0.,0.,-1.));
#6161=DIRECTION('',(0.,1.,0.));
#6162=DIRECTION('center_axis',(1.,0.,0.));
#6163=DIRECTION('ref_axis',(0.,0.,-1.));
#6164=DIRECTION('',(0.,0.,1.));
#6165=DIRECTION('center_axis',(1.,0.,0.));
#6166=DIRECTION('ref_axis',(0.,0.,-1.));
#6167=DIRECTION('',(0.,1.,0.));
#6168=DIRECTION('center_axis',(1.,0.,0.));
#6169=DIRECTION('ref_axis',(0.,0.,-1.));
#6170=DIRECTION('',(0.,0.,1.));
#6171=DIRECTION('center_axis',(0.,-1.,0.));
#6172=DIRECTION('ref_axis',(0.,0.,-1.));
#6173=DIRECTION('',(0.,0.,1.));
#6174=DIRECTION('',(1.,0.,0.));
#6175=DIRECTION('',(0.,0.,1.));
#6176=DIRECTION('',(1.,0.,0.));
#6177=DIRECTION('center_axis',(0.,-1.,0.));
#6178=DIRECTION('ref_axis',(0.,0.,-1.));
#6179=DIRECTION('',(0.,0.,1.));
#6180=DIRECTION('',(1.,0.,0.));
#6181=DIRECTION('',(0.,0.,1.));
#6182=DIRECTION('',(1.,0.,0.));
#6183=DIRECTION('center_axis',(0.,-1.,0.));
#6184=DIRECTION('ref_axis',(0.,0.,-1.));
#6185=DIRECTION('',(0.,0.,1.));
#6186=DIRECTION('',(1.,0.,0.));
#6187=DIRECTION('',(0.,0.,1.));
#6188=DIRECTION('',(1.,0.,0.));
#6189=DIRECTION('center_axis',(1.,0.,0.));
#6190=DIRECTION('ref_axis',(0.,0.,-1.));
#6191=DIRECTION('center_axis',(1.,0.,0.));
#6192=DIRECTION('ref_axis',(0.,0.,-1.));
#6193=DIRECTION('',(0.,1.,0.));
#6194=DIRECTION('',(0.,0.,1.));
#6195=DIRECTION('center_axis',(1.,0.,0.));
#6196=DIRECTION('ref_axis',(0.,0.,-1.));
#6197=DIRECTION('',(0.,1.,0.));
#6198=DIRECTION('center_axis',(1.,0.,0.));
#6199=DIRECTION('ref_axis',(0.,0.,-1.));
#6200=DIRECTION('',(0.,0.,1.));
#6201=DIRECTION('center_axis',(0.,-1.,0.));
#6202=DIRECTION('ref_axis',(0.,0.,-1.));
#6203=DIRECTION('',(0.,0.,1.));
#6204=DIRECTION('',(1.,0.,0.));
#6205=DIRECTION('',(0.,0.,1.));
#6206=DIRECTION('',(1.,0.,0.));
#6207=DIRECTION('center_axis',(0.,-1.,0.));
#6208=DIRECTION('ref_axis',(0.,0.,-1.));
#6209=DIRECTION('',(1.,0.,0.));
#6210=DIRECTION('',(1.,0.,0.));
#6211=DIRECTION('center_axis',(-2.89120579329468E-16,-1.,0.));
#6212=DIRECTION('ref_axis',(1.,-2.89120579329468E-16,0.));
#6213=DIRECTION('',(1.,0.,0.));
#6214=DIRECTION('',(0.,0.,1.));
#6215=DIRECTION('',(1.,-2.89120579329468E-16,0.));
#6216=DIRECTION('center_axis',(0.,-1.,0.));
#6217=DIRECTION('ref_axis',(0.,0.,-1.));
#6218=DIRECTION('',(1.,0.,0.));
#6219=DIRECTION('',(1.,0.,0.));
#6220=DIRECTION('center_axis',(0.,0.,-1.));
#6221=DIRECTION('ref_axis',(1.,0.,0.));
#6222=DIRECTION('',(0.,-1.,0.));
#6223=DIRECTION('',(1.,0.,0.));
#6224=DIRECTION('',(0.,1.,0.));
#6225=DIRECTION('',(0.,1.,0.));
#6226=DIRECTION('',(1.,0.,0.));
#6227=DIRECTION('',(0.,1.,0.));
#6228=DIRECTION('',(1.73472347597681E-16,1.,0.));
#6229=DIRECTION('',(1.,0.,0.));
#6230=DIRECTION('',(1.7347234759768E-16,1.,0.));
#6231=DIRECTION('',(0.,1.,0.));
#6232=DIRECTION('',(1.,0.,0.));
#6233=DIRECTION('',(0.,1.,0.));
#6234=DIRECTION('',(0.,1.,0.));
#6235=DIRECTION('',(1.,0.,0.));
#6236=DIRECTION('',(0.,-1.,0.));
#6237=DIRECTION('',(1.,0.,0.));
#6238=DIRECTION('center_axis',(0.,0.,1.));
#6239=DIRECTION('ref_axis',(1.,0.,0.));
#6240=DIRECTION('',(0.,-1.,0.));
#6241=DIRECTION('',(1.,0.,0.));
#6242=DIRECTION('',(0.,-1.,0.));
#6243=DIRECTION('center_axis',(1.,1.82602471155453E-16,0.));
#6244=DIRECTION('ref_axis',(-1.82602471155453E-16,1.,0.));
#6245=DIRECTION('',(3.16764793484742E-32,-1.7347234759768E-16,-1.));
#6246=DIRECTION('',(-1.82602471155453E-16,1.,0.));
#6247=DIRECTION('',(0.,0.,-1.));
#6248=DIRECTION('',(-1.82602471155453E-16,1.,0.));
#6249=DIRECTION('center_axis',(1.,0.,0.));
#6250=DIRECTION('ref_axis',(0.,0.,-1.));
#6251=DIRECTION('center_axis',(-1.,0.,0.));
#6252=DIRECTION('ref_axis',(0.,0.,1.));
#6253=DIRECTION('',(0.,-1.,0.));
#6254=DIRECTION('',(0.,-1.,0.));
#6255=DIRECTION('',(0.,1.7347234759768E-16,1.));
#6256=DIRECTION('',(0.,-1.,0.));
#6257=DIRECTION('center_axis',(1.,0.,0.));
#6258=DIRECTION('ref_axis',(0.,0.,-1.));
#6259=DIRECTION('',(0.,0.,1.));
#6260=DIRECTION('',(0.,-1.,0.));
#6261=DIRECTION('center_axis',(1.,0.,0.));
#6262=DIRECTION('ref_axis',(0.,0.,-1.));
#6263=DIRECTION('',(0.,0.,-1.));
#6264=DIRECTION('center_axis',(0.,1.,0.));
#6265=DIRECTION('ref_axis',(0.,0.,1.));
#6266=DIRECTION('',(0.,0.,-1.));
#6267=DIRECTION('center_axis',(0.,-1.,0.));
#6268=DIRECTION('ref_axis',(0.,0.,-1.));
#6269=DIRECTION('center_axis',(0.,-1.,0.));
#6270=DIRECTION('ref_axis',(0.,0.,-1.));
#6271=DIRECTION('center_axis',(0.,-1.,0.));
#6272=DIRECTION('ref_axis',(0.,0.,-1.));
#6273=DIRECTION('center_axis',(0.,-1.,0.));
#6274=DIRECTION('ref_axis',(0.,0.,-1.));
#6275=DIRECTION('center_axis',(0.,-1.,0.));
#6276=DIRECTION('ref_axis',(0.,0.,-1.));
#6277=DIRECTION('center_axis',(1.,0.,0.));
#6278=DIRECTION('ref_axis',(0.,0.,-1.));
#6279=DIRECTION('',(0.,-1.,0.));
#6280=DIRECTION('center_axis',(1.,0.,0.));
#6281=DIRECTION('ref_axis',(0.,0.,-1.));
#6282=DIRECTION('center_axis',(1.,0.,0.));
#6283=DIRECTION('ref_axis',(0.,0.,-1.));
#6284=DIRECTION('',(0.,-1.,0.));
#6285=DIRECTION('',(0.,0.,1.));
#6286=DIRECTION('center_axis',(1.,0.,0.));
#6287=DIRECTION('ref_axis',(0.,0.,-1.));
#6288=DIRECTION('center_axis',(0.,1.,0.));
#6289=DIRECTION('ref_axis',(0.,0.,1.));
#6290=DIRECTION('center_axis',(0.,1.,0.));
#6291=DIRECTION('ref_axis',(0.,0.,1.));
#6292=DIRECTION('center_axis',(0.,1.,0.));
#6293=DIRECTION('ref_axis',(0.,0.,1.));
#6294=DIRECTION('center_axis',(0.,1.,0.));
#6295=DIRECTION('ref_axis',(0.,0.,1.));
#6296=DIRECTION('center_axis',(0.,1.,0.));
#6297=DIRECTION('ref_axis',(0.,0.,1.));
#6298=DIRECTION('center_axis',(0.,1.,0.));
#6299=DIRECTION('ref_axis',(0.,0.,1.));
#6300=DIRECTION('center_axis',(0.,0.,-1.));
#6301=DIRECTION('ref_axis',(-1.,0.,0.));
#6302=DIRECTION('',(-1.,0.,0.));
#6303=DIRECTION('center_axis',(0.,0.,-1.));
#6304=DIRECTION('ref_axis',(-1.,0.,0.));
#6305=DIRECTION('',(-1.,0.,0.));
#6306=DIRECTION('center_axis',(0.,-1.,1.7347234759768E-16));
#6307=DIRECTION('ref_axis',(0.,-1.7347234759768E-16,-1.));
#6308=DIRECTION('center_axis',(0.,-1.,0.));
#6309=DIRECTION('ref_axis',(0.,0.,-1.));
#6310=DIRECTION('',(0.,-1.,0.));
#6311=DIRECTION('center_axis',(0.,-1.,0.));
#6312=DIRECTION('ref_axis',(0.,0.,-1.));
#6313=DIRECTION('',(0.,-1.,0.));
#6314=DIRECTION('center_axis',(0.,-1.,0.));
#6315=DIRECTION('ref_axis',(0.,0.,-1.));
#6316=DIRECTION('',(0.,-1.,0.));
#6317=DIRECTION('center_axis',(0.,-1.,0.));
#6318=DIRECTION('ref_axis',(0.,0.,-1.));
#6319=DIRECTION('',(0.,-1.,0.));
#6320=DIRECTION('center_axis',(0.,-1.,0.));
#6321=DIRECTION('ref_axis',(0.,0.,-1.));
#6322=DIRECTION('',(0.,-1.,0.));
#6323=DIRECTION('center_axis',(0.,-1.,0.));
#6324=DIRECTION('ref_axis',(0.,0.,-1.));
#6325=DIRECTION('',(1.,0.,0.));
#6326=DIRECTION('',(1.,0.,0.));
#6327=DIRECTION('center_axis',(1.,-1.7347234759768E-16,0.));
#6328=DIRECTION('ref_axis',(1.7347234759768E-16,1.,0.));
#6329=DIRECTION('center_axis',(1.,-1.7347234759768E-16,0.));
#6330=DIRECTION('ref_axis',(1.7347234759768E-16,1.,0.));
#6331=DIRECTION('',(1.7347234759768E-16,1.,0.));
#6332=DIRECTION('center_axis',(1.,0.,0.));
#6333=DIRECTION('ref_axis',(0.,0.,-1.));
#6334=DIRECTION('center_axis',(1.,0.,0.));
#6335=DIRECTION('ref_axis',(0.,0.,-1.));
#6336=DIRECTION('center_axis',(1.,0.,0.));
#6337=DIRECTION('ref_axis',(0.,0.,-1.));
#6338=DIRECTION('center_axis',(1.,0.,0.));
#6339=DIRECTION('ref_axis',(0.,0.,-1.));
#6340=DIRECTION('center_axis',(1.,-1.7347234759768E-16,0.));
#6341=DIRECTION('ref_axis',(1.7347234759768E-16,1.,0.));
#6342=DIRECTION('center_axis',(1.,-1.7347234759768E-16,0.));
#6343=DIRECTION('ref_axis',(1.7347234759768E-16,1.,0.));
#6344=DIRECTION('center_axis',(1.,0.,0.));
#6345=DIRECTION('ref_axis',(0.,0.,-1.));
#6346=DIRECTION('center_axis',(1.,0.,0.));
#6347=DIRECTION('ref_axis',(0.,0.,-1.));
#6348=DIRECTION('center_axis',(-1.,1.7347234759768E-16,0.));
#6349=DIRECTION('ref_axis',(-1.7347234759768E-16,-1.,0.));
#6350=DIRECTION('center_axis',(-1.,1.7347234759768E-16,0.));
#6351=DIRECTION('ref_axis',(-1.7347234759768E-16,-1.,0.));
#6352=DIRECTION('',(0.,0.,1.));
#6353=DIRECTION('',(-1.7347234759768E-16,-1.,0.));
#6354=DIRECTION('center_axis',(1.44560289664734E-16,1.,0.));
#6355=DIRECTION('ref_axis',(-1.,1.44560289664734E-16,0.));
#6356=DIRECTION('',(1.,0.,0.));
#6357=DIRECTION('',(0.,0.,1.));
#6358=DIRECTION('',(-1.,1.44560289664734E-16,0.));
#6359=DIRECTION('center_axis',(-1.,0.,0.));
#6360=DIRECTION('ref_axis',(0.,0.,1.));
#6361=DIRECTION('center_axis',(-1.,0.,0.));
#6362=DIRECTION('ref_axis',(0.,0.,1.));
#6363=DIRECTION('',(0.,-1.,0.));
#6364=DIRECTION('center_axis',(1.,0.,0.));
#6365=DIRECTION('ref_axis',(0.,0.,-1.));
#6366=DIRECTION('center_axis',(1.,0.,0.));
#6367=DIRECTION('ref_axis',(0.,0.,-1.));
#6368=DIRECTION('center_axis',(1.,-1.73472347597681E-16,0.));
#6369=DIRECTION('ref_axis',(1.73472347597681E-16,1.,0.));
#6370=DIRECTION('center_axis',(1.,-1.73472347597681E-16,0.));
#6371=DIRECTION('ref_axis',(1.73472347597681E-16,1.,0.));
#6372=DIRECTION('center_axis',(1.,0.,0.));
#6373=DIRECTION('ref_axis',(0.,0.,-1.));
#6374=DIRECTION('center_axis',(1.,0.,0.));
#6375=DIRECTION('ref_axis',(0.,0.,-1.));
#6376=DIRECTION('center_axis',(1.,0.,0.));
#6377=DIRECTION('ref_axis',(0.,0.,-1.));
#6378=DIRECTION('center_axis',(1.,0.,0.));
#6379=DIRECTION('ref_axis',(0.,0.,-1.));
#6380=DIRECTION('center_axis',(0.,0.,-1.));
#6381=DIRECTION('ref_axis',(1.,0.,0.));
#6382=DIRECTION('',(1.,0.,0.));
#6383=DIRECTION('',(1.,0.,0.));
#6384=DIRECTION('',(1.,0.,0.));
#6385=DIRECTION('',(1.,0.,0.));
#6386=DIRECTION('',(1.,0.,0.));
#6387=DIRECTION('center_axis',(1.,0.,0.));
#6388=DIRECTION('ref_axis',(0.,5.66553889764798E-16,1.));
#6389=DIRECTION('center_axis',(1.,0.,0.));
#6390=DIRECTION('ref_axis',(0.,0.,-1.));
#6391=DIRECTION('',(1.,0.,0.));
#6392=DIRECTION('center_axis',(1.,0.,0.));
#6393=DIRECTION('ref_axis',(0.,0.,-1.));
#6394=DIRECTION('',(1.,0.,0.));
#6395=DIRECTION('center_axis',(1.,-1.7347234759768E-16,0.));
#6396=DIRECTION('ref_axis',(1.7347234759768E-16,1.,0.));
#6397=DIRECTION('',(1.,0.,0.));
#6398=DIRECTION('center_axis',(1.,0.,0.));
#6399=DIRECTION('ref_axis',(0.,0.,-1.));
#6400=DIRECTION('',(1.,0.,0.));
#6401=DIRECTION('',(1.,0.,0.));
#6402=DIRECTION('center_axis',(1.,0.,0.));
#6403=DIRECTION('ref_axis',(0.,0.,-1.));
#6404=DIRECTION('',(1.,0.,0.));
#6405=DIRECTION('center_axis',(1.,0.,0.));
#6406=DIRECTION('ref_axis',(0.,0.,-1.));
#6407=DIRECTION('',(1.,0.,0.));
#6408=DIRECTION('center_axis',(1.,-1.7347234759768E-16,0.));
#6409=DIRECTION('ref_axis',(1.7347234759768E-16,1.,0.));
#6410=DIRECTION('',(1.,0.,0.));
#6411=DIRECTION('center_axis',(1.,0.,0.));
#6412=DIRECTION('ref_axis',(0.,0.,-1.));
#6413=DIRECTION('',(1.,0.,0.));
#6414=DIRECTION('center_axis',(-1.,1.7347234759768E-16,0.));
#6415=DIRECTION('ref_axis',(-1.7347234759768E-16,-1.,0.));
#6416=DIRECTION('',(1.,0.,0.));
#6417=DIRECTION('center_axis',(-1.,0.,0.));
#6418=DIRECTION('ref_axis',(0.,0.,1.));
#6419=DIRECTION('',(1.,0.,0.));
#6420=DIRECTION('center_axis',(1.,0.,0.));
#6421=DIRECTION('ref_axis',(0.,0.,-1.));
#6422=DIRECTION('',(1.,0.,0.));
#6423=DIRECTION('center_axis',(1.,-1.73472347597681E-16,0.));
#6424=DIRECTION('ref_axis',(1.73472347597681E-16,1.,0.));
#6425=DIRECTION('center_axis',(1.,0.,0.));
#6426=DIRECTION('ref_axis',(0.,0.,-1.));
#6427=DIRECTION('',(1.,0.,0.));
#6428=DIRECTION('center_axis',(1.,0.,0.));
#6429=DIRECTION('ref_axis',(0.,0.,-1.));
#6430=DIRECTION('',(1.,0.,0.));
#6431=DIRECTION('',(1.,0.,0.));
#6432=DIRECTION('center_axis',(1.,0.,0.));
#6433=DIRECTION('ref_axis',(0.,0.,-1.));
#6434=DIRECTION('',(1.,0.,0.));
#6435=DIRECTION('center_axis',(1.,0.,0.));
#6436=DIRECTION('ref_axis',(0.,0.,-1.));
#6437=DIRECTION('center_axis',(1.,0.,0.));
#6438=DIRECTION('ref_axis',(0.,0.,-1.));
#6439=DIRECTION('center_axis',(1.,0.,0.));
#6440=DIRECTION('ref_axis',(0.,0.,-1.));
#6441=DIRECTION('center_axis',(1.,0.,0.));
#6442=DIRECTION('ref_axis',(0.,0.,-1.));
#6443=DIRECTION('',(0.,0.,1.));
#6444=DIRECTION('center_axis',(0.,-1.,0.));
#6445=DIRECTION('ref_axis',(0.,0.,-1.));
#6446=DIRECTION('',(0.,0.,1.));
#6447=DIRECTION('center_axis',(1.,0.,0.));
#6448=DIRECTION('ref_axis',(0.,0.,-1.));
#6449=DIRECTION('center_axis',(1.,0.,0.));
#6450=DIRECTION('ref_axis',(0.,0.,-1.));
#6451=DIRECTION('center_axis',(1.,0.,0.));
#6452=DIRECTION('ref_axis',(0.,0.,-1.));
#6453=DIRECTION('center_axis',(0.,-1.,0.));
#6454=DIRECTION('ref_axis',(0.,0.,-1.));
#6455=DIRECTION('',(0.,0.,1.));
#6456=DIRECTION('',(0.,0.,1.));
#6457=DIRECTION('center_axis',(1.,0.,0.));
#6458=DIRECTION('ref_axis',(0.,0.,-1.));
#6459=DIRECTION('center_axis',(1.,0.,0.));
#6460=DIRECTION('ref_axis',(0.,0.,-1.));
#6461=DIRECTION('center_axis',(1.,0.,0.));
#6462=DIRECTION('ref_axis',(0.,0.,-1.));
#6463=DIRECTION('center_axis',(1.,0.,0.));
#6464=DIRECTION('ref_axis',(0.,0.,-1.));
#6465=DIRECTION('center_axis',(1.,0.,0.));
#6466=DIRECTION('ref_axis',(0.,0.,-1.));
#6467=DIRECTION('center_axis',(1.,0.,0.));
#6468=DIRECTION('ref_axis',(0.,0.,-1.));
#6469=DIRECTION('center_axis',(1.,-1.73472347597681E-16,0.));
#6470=DIRECTION('ref_axis',(1.73472347597681E-16,1.,0.));
#6471=DIRECTION('center_axis',(1.,-1.73472347597681E-16,0.));
#6472=DIRECTION('ref_axis',(1.73472347597681E-16,1.,0.));
#6473=DIRECTION('center_axis',(1.,-1.73472347597681E-16,0.));
#6474=DIRECTION('ref_axis',(1.73472347597681E-16,1.,0.));
#6475=DIRECTION('',(0.,0.,1.));
#6476=DIRECTION('center_axis',(0.,-1.,0.));
#6477=DIRECTION('ref_axis',(0.,0.,-1.));
#6478=DIRECTION('',(0.,0.,1.));
#6479=DIRECTION('center_axis',(1.,0.,0.));
#6480=DIRECTION('ref_axis',(0.,0.,-1.));
#6481=DIRECTION('center_axis',(1.,0.,0.));
#6482=DIRECTION('ref_axis',(0.,0.,-1.));
#6483=DIRECTION('center_axis',(1.,0.,0.));
#6484=DIRECTION('ref_axis',(0.,0.,-1.));
#6485=DIRECTION('center_axis',(-1.,0.,0.));
#6486=DIRECTION('ref_axis',(0.,0.,1.));
#6487=DIRECTION('center_axis',(-1.,0.,0.));
#6488=DIRECTION('ref_axis',(0.,0.,1.));
#6489=DIRECTION('center_axis',(-1.,0.,0.));
#6490=DIRECTION('ref_axis',(0.,0.,1.));
#6491=DIRECTION('',(0.,0.,1.));
#6492=DIRECTION('center_axis',(1.44560289664734E-16,1.,0.));
#6493=DIRECTION('ref_axis',(-1.,1.44560289664734E-16,0.));
#6494=DIRECTION('',(0.,0.,1.));
#6495=DIRECTION('center_axis',(-1.,1.7347234759768E-16,0.));
#6496=DIRECTION('ref_axis',(-1.7347234759768E-16,-1.,0.));
#6497=DIRECTION('center_axis',(-1.,1.7347234759768E-16,0.));
#6498=DIRECTION('ref_axis',(-1.7347234759768E-16,-1.,0.));
#6499=DIRECTION('center_axis',(-1.,1.7347234759768E-16,0.));
#6500=DIRECTION('ref_axis',(-1.7347234759768E-16,-1.,0.));
#6501=DIRECTION('center_axis',(1.,0.,0.));
#6502=DIRECTION('ref_axis',(0.,0.,-1.));
#6503=DIRECTION('center_axis',(1.,0.,0.));
#6504=DIRECTION('ref_axis',(0.,0.,-1.));
#6505=DIRECTION('center_axis',(1.,0.,0.));
#6506=DIRECTION('ref_axis',(0.,0.,-1.));
#6507=DIRECTION('',(0.,0.,1.));
#6508=DIRECTION('center_axis',(0.,-1.,0.));
#6509=DIRECTION('ref_axis',(0.,0.,-1.));
#6510=DIRECTION('',(0.,0.,1.));
#6511=DIRECTION('center_axis',(1.,-1.7347234759768E-16,0.));
#6512=DIRECTION('ref_axis',(1.7347234759768E-16,1.,0.));
#6513=DIRECTION('center_axis',(1.,-1.7347234759768E-16,0.));
#6514=DIRECTION('ref_axis',(1.7347234759768E-16,1.,0.));
#6515=DIRECTION('center_axis',(1.,-1.7347234759768E-16,0.));
#6516=DIRECTION('ref_axis',(1.7347234759768E-16,1.,0.));
#6517=DIRECTION('center_axis',(1.,0.,0.));
#6518=DIRECTION('ref_axis',(0.,0.,-1.));
#6519=DIRECTION('center_axis',(1.,0.,0.));
#6520=DIRECTION('ref_axis',(0.,0.,-1.));
#6521=DIRECTION('center_axis',(1.,0.,0.));
#6522=DIRECTION('ref_axis',(0.,0.,-1.));
#6523=DIRECTION('',(0.,0.,1.));
#6524=DIRECTION('center_axis',(0.,-1.,0.));
#6525=DIRECTION('ref_axis',(0.,0.,-1.));
#6526=DIRECTION('',(0.,0.,1.));
#6527=DIRECTION('center_axis',(1.,0.,0.));
#6528=DIRECTION('ref_axis',(0.,0.,-1.));
#6529=DIRECTION('center_axis',(1.,0.,0.));
#6530=DIRECTION('ref_axis',(0.,0.,-1.));
#6531=DIRECTION('center_axis',(1.,0.,0.));
#6532=DIRECTION('ref_axis',(0.,0.,-1.));
#6533=DIRECTION('center_axis',(-2.89120579329468E-16,-1.,0.));
#6534=DIRECTION('ref_axis',(1.,-2.89120579329468E-16,0.));
#6535=DIRECTION('',(0.,0.,1.));
#6536=DIRECTION('',(0.,0.,1.));
#6537=DIRECTION('center_axis',(1.,0.,0.));
#6538=DIRECTION('ref_axis',(0.,0.,-1.));
#6539=DIRECTION('center_axis',(1.,0.,0.));
#6540=DIRECTION('ref_axis',(0.,0.,-1.));
#6541=DIRECTION('center_axis',(1.,0.,0.));
#6542=DIRECTION('ref_axis',(0.,0.,-1.));
#6543=DIRECTION('center_axis',(1.,-1.7347234759768E-16,0.));
#6544=DIRECTION('ref_axis',(1.7347234759768E-16,1.,0.));
#6545=DIRECTION('center_axis',(1.,-1.7347234759768E-16,0.));
#6546=DIRECTION('ref_axis',(1.7347234759768E-16,1.,0.));
#6547=DIRECTION('center_axis',(1.,-1.7347234759768E-16,0.));
#6548=DIRECTION('ref_axis',(1.7347234759768E-16,1.,0.));
#6549=DIRECTION('center_axis',(0.,-1.,0.));
#6550=DIRECTION('ref_axis',(0.,0.,-1.));
#6551=DIRECTION('',(0.,0.,1.));
#6552=DIRECTION('',(0.,0.,1.));
#6553=DIRECTION('center_axis',(1.,0.,0.));
#6554=DIRECTION('ref_axis',(0.,0.,-1.));
#6555=DIRECTION('center_axis',(1.,0.,0.));
#6556=DIRECTION('ref_axis',(0.,0.,-1.));
#6557=DIRECTION('center_axis',(1.,0.,0.));
#6558=DIRECTION('ref_axis',(0.,0.,-1.));
#6559=DIRECTION('center_axis',(1.,0.,0.));
#6560=DIRECTION('ref_axis',(0.,0.,-1.));
#6561=DIRECTION('center_axis',(1.,0.,0.));
#6562=DIRECTION('ref_axis',(0.,0.,-1.));
#6563=DIRECTION('center_axis',(1.,0.,0.));
#6564=DIRECTION('ref_axis',(0.,0.,-1.));
#6565=DIRECTION('center_axis',(1.,0.,0.));
#6566=DIRECTION('ref_axis',(0.,0.,-1.));
#6567=DIRECTION('',(1.,0.,0.));
#6568=DIRECTION('center_axis',(-1.,5.78241158658936E-16,0.));
#6569=DIRECTION('ref_axis',(-5.78241158658936E-16,-1.,0.));
#6570=DIRECTION('center_axis',(1.,0.,0.));
#6571=DIRECTION('ref_axis',(0.,0.,-1.));
#6572=DIRECTION('',(1.,0.,0.));
#6573=DIRECTION('center_axis',(-1.,0.,0.));
#6574=DIRECTION('ref_axis',(0.,0.,1.));
#6575=DIRECTION('center_axis',(1.,0.,0.));
#6576=DIRECTION('ref_axis',(0.,0.,-1.));
#6577=DIRECTION('',(1.,0.,0.));
#6578=DIRECTION('center_axis',(-1.,0.,0.));
#6579=DIRECTION('ref_axis',(0.,0.,1.));
#6580=DIRECTION('center_axis',(1.,0.,0.));
#6581=DIRECTION('ref_axis',(0.,0.,-1.));
#6582=DIRECTION('',(1.,0.,0.));
#6583=DIRECTION('center_axis',(1.,0.,0.));
#6584=DIRECTION('ref_axis',(0.,0.,-1.));
#6585=DIRECTION('center_axis',(1.,0.,0.));
#6586=DIRECTION('ref_axis',(0.,0.,-1.));
#6587=DIRECTION('',(1.,0.,0.));
#6588=DIRECTION('center_axis',(1.,-2.89120579329468E-16,0.));
#6589=DIRECTION('ref_axis',(2.89120579329468E-16,1.,0.));
#6590=DIRECTION('center_axis',(1.,0.,0.));
#6591=DIRECTION('ref_axis',(0.,0.,-1.));
#6592=DIRECTION('',(1.,0.,0.));
#6593=DIRECTION('center_axis',(1.,-2.89120579329468E-16,0.));
#6594=DIRECTION('ref_axis',(2.89120579329468E-16,1.,0.));
#6595=DIRECTION('center_axis',(1.,0.,0.));
#6596=DIRECTION('ref_axis',(0.,0.,-1.));
#6597=DIRECTION('',(1.,0.,0.));
#6598=DIRECTION('center_axis',(1.,0.,0.));
#6599=DIRECTION('ref_axis',(0.,0.,-1.));
#6600=DIRECTION('center_axis',(1.,0.,0.));
#6601=DIRECTION('ref_axis',(0.,0.,-1.));
#6602=DIRECTION('',(1.,0.,0.));
#6603=DIRECTION('center_axis',(-1.,0.,0.));
#6604=DIRECTION('ref_axis',(0.,0.,1.));
#6605=DIRECTION('center_axis',(1.,0.,0.));
#6606=DIRECTION('ref_axis',(0.,0.,-1.));
#6607=DIRECTION('center_axis',(1.,0.,0.));
#6608=DIRECTION('ref_axis',(0.,0.,-1.));
#6609=DIRECTION('',(0.,0.,-1.));
#6610=DIRECTION('',(0.,-1.,0.));
#6611=DIRECTION('center_axis',(0.,1.,0.));
#6612=DIRECTION('ref_axis',(0.,0.,1.));
#6613=DIRECTION('',(-1.,0.,0.));
#6614=DIRECTION('',(0.,0.,-1.));
#6615=DIRECTION('',(1.,0.,0.));
#6616=DIRECTION('center_axis',(1.,0.,0.));
#6617=DIRECTION('ref_axis',(0.,0.,-1.));
#6618=DIRECTION('center_axis',(1.,0.,0.));
#6619=DIRECTION('ref_axis',(0.,0.,-1.));
#6620=DIRECTION('',(0.,-1.,0.));
#6621=DIRECTION('center_axis',(0.,1.,0.));
#6622=DIRECTION('ref_axis',(0.,0.,1.));
#6623=DIRECTION('',(-1.,0.,0.));
#6624=DIRECTION('',(0.,0.,-1.));
#6625=DIRECTION('',(1.,0.,0.));
#6626=DIRECTION('center_axis',(1.,0.,0.));
#6627=DIRECTION('ref_axis',(0.,0.,-1.));
#6628=DIRECTION('center_axis',(1.,0.,0.));
#6629=DIRECTION('ref_axis',(0.,0.,-1.));
#6630=DIRECTION('',(0.,-1.,0.));
#6631=DIRECTION('center_axis',(-1.,0.,0.));
#6632=DIRECTION('ref_axis',(0.,0.,1.));
#6633=DIRECTION('center_axis',(-1.,0.,0.));
#6634=DIRECTION('ref_axis',(0.,0.,1.));
#6635=DIRECTION('center_axis',(1.,0.,0.));
#6636=DIRECTION('ref_axis',(0.,0.,-1.));
#6637=DIRECTION('center_axis',(1.,0.,0.));
#6638=DIRECTION('ref_axis',(0.,0.,-1.));
#6639=DIRECTION('',(0.,0.,-1.));
#6640=DIRECTION('',(0.,-1.,0.));
#6641=DIRECTION('center_axis',(-2.89120579329468E-16,1.,0.));
#6642=DIRECTION('ref_axis',(-1.,-2.89120579329468E-16,0.));
#6643=DIRECTION('',(-1.,0.,0.));
#6644=DIRECTION('',(1.,2.89120579329468E-16,0.));
#6645=DIRECTION('center_axis',(1.,0.,0.));
#6646=DIRECTION('ref_axis',(0.,0.,-1.));
#6647=DIRECTION('center_axis',(1.,0.,0.));
#6648=DIRECTION('ref_axis',(0.,0.,-1.));
#6649=DIRECTION('',(0.,0.,-1.));
#6650=DIRECTION('',(0.,-1.,0.));
#6651=DIRECTION('center_axis',(0.,1.,0.));
#6652=DIRECTION('ref_axis',(0.,0.,1.));
#6653=DIRECTION('',(-1.,0.,0.));
#6654=DIRECTION('',(0.,0.,-1.));
#6655=DIRECTION('',(1.,0.,0.));
#6656=DIRECTION('center_axis',(1.,0.,0.));
#6657=DIRECTION('ref_axis',(0.,0.,-1.));
#6658=DIRECTION('center_axis',(1.,0.,0.));
#6659=DIRECTION('ref_axis',(0.,0.,-1.));
#6660=DIRECTION('',(0.,-1.,0.));
#6661=DIRECTION('center_axis',(0.,1.,0.));
#6662=DIRECTION('ref_axis',(0.,0.,1.));
#6663=DIRECTION('',(-1.,0.,0.));
#6664=DIRECTION('center_axis',(0.,1.,0.));
#6665=DIRECTION('ref_axis',(0.,0.,1.));
#6666=DIRECTION('',(-1.,0.,0.));
#6667=DIRECTION('center_axis',(0.,1.,0.));
#6668=DIRECTION('ref_axis',(0.,0.,1.));
#6669=DIRECTION('',(-1.,0.,0.));
#6670=DIRECTION('center_axis',(0.,0.,1.));
#6671=DIRECTION('ref_axis',(1.,0.,0.));
#6672=DIRECTION('',(-1.,0.,0.));
#6673=DIRECTION('',(-1.,0.,0.));
#6674=DIRECTION('',(-1.,0.,0.));
#6675=DIRECTION('',(-1.,0.,0.));
#6676=DIRECTION('',(-1.,0.,0.));
#6677=DIRECTION('center_axis',(-1.,0.,0.));
#6678=DIRECTION('ref_axis',(0.,5.66553889764798E-16,-1.));
#6679=DIRECTION('center_axis',(1.,0.,0.));
#6680=DIRECTION('ref_axis',(0.,0.,-1.));
#6681=DIRECTION('',(-1.,0.,0.));
#6682=DIRECTION('center_axis',(1.,0.,0.));
#6683=DIRECTION('ref_axis',(0.,0.,-1.));
#6684=DIRECTION('',(-1.,0.,0.));
#6685=DIRECTION('',(-1.,0.,0.));
#6686=DIRECTION('center_axis',(1.,0.,0.));
#6687=DIRECTION('ref_axis',(0.,0.,-1.));
#6688=DIRECTION('',(-1.,0.,0.));
#6689=DIRECTION('center_axis',(1.,0.,0.));
#6690=DIRECTION('ref_axis',(0.,0.,-1.));
#6691=DIRECTION('',(-1.,0.,0.));
#6692=DIRECTION('center_axis',(1.,1.7347234759768E-16,0.));
#6693=DIRECTION('ref_axis',(-1.7347234759768E-16,1.,0.));
#6694=DIRECTION('',(-1.,0.,0.));
#6695=DIRECTION('center_axis',(1.,0.,0.));
#6696=DIRECTION('ref_axis',(0.,0.,-1.));
#6697=DIRECTION('',(-1.,0.,0.));
#6698=DIRECTION('center_axis',(-1.,-1.7347234759768E-16,0.));
#6699=DIRECTION('ref_axis',(1.7347234759768E-16,-1.,0.));
#6700=DIRECTION('',(-1.,0.,0.));
#6701=DIRECTION('center_axis',(-1.,0.,0.));
#6702=DIRECTION('ref_axis',(0.,0.,1.));
#6703=DIRECTION('',(-1.,0.,0.));
#6704=DIRECTION('center_axis',(1.,0.,0.));
#6705=DIRECTION('ref_axis',(0.,0.,-1.));
#6706=DIRECTION('',(-1.,0.,0.));
#6707=DIRECTION('center_axis',(1.,1.7347234759768E-16,0.));
#6708=DIRECTION('ref_axis',(-1.7347234759768E-16,1.,0.));
#6709=DIRECTION('center_axis',(1.,0.,0.));
#6710=DIRECTION('ref_axis',(0.,0.,-1.));
#6711=DIRECTION('',(-1.,0.,0.));
#6712=DIRECTION('center_axis',(1.,0.,0.));
#6713=DIRECTION('ref_axis',(0.,0.,-1.));
#6714=DIRECTION('',(-1.,0.,0.));
#6715=DIRECTION('',(-1.,0.,0.));
#6716=DIRECTION('center_axis',(1.,0.,0.));
#6717=DIRECTION('ref_axis',(0.,0.,-1.));
#6718=DIRECTION('',(-1.,0.,0.));
#6719=DIRECTION('center_axis',(1.,0.,0.));
#6720=DIRECTION('ref_axis',(0.,0.,-1.));
#6721=DIRECTION('center_axis',(1.,0.,0.));
#6722=DIRECTION('ref_axis',(0.,0.,-1.));
#6723=DIRECTION('',(-1.,0.,0.));
#6724=DIRECTION('center_axis',(1.,0.,0.));
#6725=DIRECTION('ref_axis',(0.,0.,-1.));
#6726=DIRECTION('',(-1.,0.,0.));
#6727=DIRECTION('center_axis',(0.,1.,0.));
#6728=DIRECTION('ref_axis',(0.,0.,1.));
#6729=DIRECTION('',(0.,0.,-1.));
#6730=DIRECTION('',(0.,0.,-1.));
#6731=DIRECTION('center_axis',(1.,0.,0.));
#6732=DIRECTION('ref_axis',(0.,0.,-1.));
#6733=DIRECTION('center_axis',(1.,0.,0.));
#6734=DIRECTION('ref_axis',(0.,0.,-1.));
#6735=DIRECTION('',(0.,0.,-1.));
#6736=DIRECTION('center_axis',(1.,0.,0.));
#6737=DIRECTION('ref_axis',(0.,0.,-1.));
#6738=DIRECTION('center_axis',(0.,1.,0.));
#6739=DIRECTION('ref_axis',(0.,0.,1.));
#6740=DIRECTION('',(0.,0.,-1.));
#6741=DIRECTION('',(1.,0.,0.));
#6742=DIRECTION('',(-1.,0.,0.));
#6743=DIRECTION('center_axis',(1.,0.,0.));
#6744=DIRECTION('ref_axis',(0.,0.,-1.));
#6745=DIRECTION('center_axis',(1.,0.,0.));
#6746=DIRECTION('ref_axis',(0.,0.,-1.));
#6747=DIRECTION('center_axis',(1.,0.,0.));
#6748=DIRECTION('ref_axis',(0.,0.,-1.));
#6749=DIRECTION('center_axis',(0.,1.,0.));
#6750=DIRECTION('ref_axis',(0.,0.,1.));
#6751=DIRECTION('',(0.,0.,-1.));
#6752=DIRECTION('',(1.,0.,0.));
#6753=DIRECTION('',(0.,0.,-1.));
#6754=DIRECTION('',(1.,0.,0.));
#6755=DIRECTION('center_axis',(1.,0.,0.));
#6756=DIRECTION('ref_axis',(0.,0.,-1.));
#6757=DIRECTION('center_axis',(1.,0.,0.));
#6758=DIRECTION('ref_axis',(0.,0.,-1.));
#6759=DIRECTION('',(0.,0.,-1.));
#6760=DIRECTION('center_axis',(1.,0.,0.));
#6761=DIRECTION('ref_axis',(0.,0.,-1.));
#6762=DIRECTION('center_axis',(0.,1.,0.));
#6763=DIRECTION('ref_axis',(0.,0.,1.));
#6764=DIRECTION('',(0.,0.,-1.));
#6765=DIRECTION('center_axis',(1.,0.,0.));
#6766=DIRECTION('ref_axis',(0.,0.,-1.));
#6767=DIRECTION('center_axis',(1.,0.,0.));
#6768=DIRECTION('ref_axis',(0.,0.,-1.));
#6769=DIRECTION('center_axis',(1.,0.,0.));
#6770=DIRECTION('ref_axis',(0.,0.,-1.));
#6771=DIRECTION('center_axis',(0.,1.,0.));
#6772=DIRECTION('ref_axis',(0.,0.,1.));
#6773=DIRECTION('',(0.,0.,-1.));
#6774=DIRECTION('',(0.,0.,-1.));
#6775=DIRECTION('center_axis',(1.,0.,0.));
#6776=DIRECTION('ref_axis',(0.,0.,-1.));
#6777=DIRECTION('center_axis',(1.,0.,0.));
#6778=DIRECTION('ref_axis',(0.,0.,-1.));
#6779=DIRECTION('',(0.,0.,-1.));
#6780=DIRECTION('center_axis',(1.,0.,0.));
#6781=DIRECTION('ref_axis',(0.,0.,-1.));
#6782=DIRECTION('center_axis',(0.,1.,0.));
#6783=DIRECTION('ref_axis',(0.,0.,1.));
#6784=DIRECTION('',(0.,0.,-1.));
#6785=DIRECTION('',(1.,0.,0.));
#6786=DIRECTION('',(-1.,0.,0.));
#6787=DIRECTION('center_axis',(1.,0.,0.));
#6788=DIRECTION('ref_axis',(0.,0.,-1.));
#6789=DIRECTION('center_axis',(1.,0.,0.));
#6790=DIRECTION('ref_axis',(0.,0.,-1.));
#6791=DIRECTION('center_axis',(1.,0.,0.));
#6792=DIRECTION('ref_axis',(0.,0.,-1.));
#6793=DIRECTION('center_axis',(0.,1.,0.));
#6794=DIRECTION('ref_axis',(0.,0.,1.));
#6795=DIRECTION('',(0.,0.,-1.));
#6796=DIRECTION('',(1.,0.,0.));
#6797=DIRECTION('',(0.,0.,-1.));
#6798=DIRECTION('',(1.,0.,0.));
#6799=DIRECTION('center_axis',(1.,1.7347234759768E-16,0.));
#6800=DIRECTION('ref_axis',(-1.7347234759768E-16,1.,0.));
#6801=DIRECTION('center_axis',(1.,1.7347234759768E-16,0.));
#6802=DIRECTION('ref_axis',(-1.7347234759768E-16,1.,0.));
#6803=DIRECTION('',(0.,0.,-1.));
#6804=DIRECTION('center_axis',(1.,1.7347234759768E-16,0.));
#6805=DIRECTION('ref_axis',(-1.7347234759768E-16,1.,0.));
#6806=DIRECTION('center_axis',(-2.89120579329468E-16,1.,0.));
#6807=DIRECTION('ref_axis',(-1.,-2.89120579329468E-16,0.));
#6808=DIRECTION('',(0.,0.,-1.));
#6809=DIRECTION('center_axis',(1.,0.,0.));
#6810=DIRECTION('ref_axis',(0.,0.,-1.));
#6811=DIRECTION('center_axis',(1.,0.,0.));
#6812=DIRECTION('ref_axis',(0.,0.,-1.));
#6813=DIRECTION('center_axis',(1.,0.,0.));
#6814=DIRECTION('ref_axis',(0.,0.,-1.));
#6815=DIRECTION('center_axis',(0.,-1.,0.));
#6816=DIRECTION('ref_axis',(0.,0.,-1.));
#6817=DIRECTION('',(0.,0.,-1.));
#6818=DIRECTION('',(-1.,0.,0.));
#6819=DIRECTION('',(0.,0.,-1.));
#6820=DIRECTION('',(1.,0.,0.));
#6821=DIRECTION('center_axis',(-1.,0.,0.));
#6822=DIRECTION('ref_axis',(0.,0.,1.));
#6823=DIRECTION('center_axis',(-1.,0.,0.));
#6824=DIRECTION('ref_axis',(0.,0.,1.));
#6825=DIRECTION('',(0.,0.,-1.));
#6826=DIRECTION('center_axis',(-1.,0.,0.));
#6827=DIRECTION('ref_axis',(0.,0.,1.));
#6828=DIRECTION('center_axis',(0.,-1.,0.));
#6829=DIRECTION('ref_axis',(0.,0.,-1.));
#6830=DIRECTION('',(0.,0.,-1.));
#6831=DIRECTION('center_axis',(-1.,-1.7347234759768E-16,0.));
#6832=DIRECTION('ref_axis',(1.7347234759768E-16,-1.,0.));
#6833=DIRECTION('center_axis',(-1.,-1.7347234759768E-16,0.));
#6834=DIRECTION('ref_axis',(1.7347234759768E-16,-1.,0.));
#6835=DIRECTION('center_axis',(-1.,-1.7347234759768E-16,0.));
#6836=DIRECTION('ref_axis',(1.7347234759768E-16,-1.,0.));
#6837=DIRECTION('center_axis',(0.,1.,0.));
#6838=DIRECTION('ref_axis',(0.,0.,1.));
#6839=DIRECTION('',(0.,0.,-1.));
#6840=DIRECTION('',(1.,0.,0.));
#6841=DIRECTION('',(0.,0.,-1.));
#6842=DIRECTION('',(1.,0.,0.));
#6843=DIRECTION('center_axis',(1.,0.,0.));
#6844=DIRECTION('ref_axis',(0.,0.,-1.));
#6845=DIRECTION('center_axis',(1.,0.,0.));
#6846=DIRECTION('ref_axis',(0.,0.,-1.));
#6847=DIRECTION('',(0.,0.,-1.));
#6848=DIRECTION('center_axis',(1.,0.,0.));
#6849=DIRECTION('ref_axis',(0.,0.,-1.));
#6850=DIRECTION('center_axis',(0.,1.,0.));
#6851=DIRECTION('ref_axis',(0.,0.,1.));
#6852=DIRECTION('',(0.,0.,-1.));
#6853=DIRECTION('center_axis',(1.,1.7347234759768E-16,0.));
#6854=DIRECTION('ref_axis',(-1.7347234759768E-16,1.,0.));
#6855=DIRECTION('center_axis',(1.,1.7347234759768E-16,0.));
#6856=DIRECTION('ref_axis',(-1.7347234759768E-16,1.,0.));
#6857=DIRECTION('center_axis',(1.,1.7347234759768E-16,0.));
#6858=DIRECTION('ref_axis',(-1.7347234759768E-16,1.,0.));
#6859=DIRECTION('center_axis',(0.,1.,0.));
#6860=DIRECTION('ref_axis',(0.,0.,1.));
#6861=DIRECTION('',(0.,0.,-1.));
#6862=DIRECTION('',(1.,0.,0.));
#6863=DIRECTION('',(0.,0.,-1.));
#6864=DIRECTION('',(1.,0.,0.));
#6865=DIRECTION('center_axis',(1.,0.,0.));
#6866=DIRECTION('ref_axis',(0.,0.,-1.));
#6867=DIRECTION('center_axis',(1.,0.,0.));
#6868=DIRECTION('ref_axis',(0.,0.,-1.));
#6869=DIRECTION('',(0.,0.,-1.));
#6870=DIRECTION('center_axis',(1.,0.,0.));
#6871=DIRECTION('ref_axis',(0.,0.,-1.));
#6872=DIRECTION('center_axis',(0.,1.,0.));
#6873=DIRECTION('ref_axis',(0.,0.,1.));
#6874=DIRECTION('',(0.,0.,-1.));
#6875=DIRECTION('center_axis',(1.,0.,0.));
#6876=DIRECTION('ref_axis',(0.,0.,-1.));
#6877=DIRECTION('center_axis',(1.,0.,0.));
#6878=DIRECTION('ref_axis',(0.,0.,-1.));
#6879=DIRECTION('center_axis',(1.,0.,0.));
#6880=DIRECTION('ref_axis',(0.,0.,-1.));
#6881=DIRECTION('center_axis',(0.,1.,0.));
#6882=DIRECTION('ref_axis',(0.,0.,1.));
#6883=DIRECTION('',(0.,0.,-1.));
#6884=DIRECTION('',(0.,0.,-1.));
#6885=DIRECTION('center_axis',(1.,0.,0.));
#6886=DIRECTION('ref_axis',(0.,0.,-1.));
#6887=DIRECTION('center_axis',(1.,0.,0.));
#6888=DIRECTION('ref_axis',(0.,0.,-1.));
#6889=DIRECTION('',(0.,0.,-1.));
#6890=DIRECTION('center_axis',(1.,0.,0.));
#6891=DIRECTION('ref_axis',(0.,0.,-1.));
#6892=DIRECTION('center_axis',(-5.78241158658936E-16,1.,0.));
#6893=DIRECTION('ref_axis',(-1.,-5.78241158658936E-16,0.));
#6894=DIRECTION('',(0.,0.,-1.));
#6895=DIRECTION('',(1.,5.78241158658936E-16,0.));
#6896=DIRECTION('',(-1.,-5.78241158658936E-16,0.));
#6897=DIRECTION('center_axis',(1.,0.,0.));
#6898=DIRECTION('ref_axis',(0.,0.,-1.));
#6899=DIRECTION('center_axis',(1.,0.,0.));
#6900=DIRECTION('ref_axis',(0.,0.,-1.));
#6901=DIRECTION('center_axis',(1.,0.,0.));
#6902=DIRECTION('ref_axis',(0.,0.,-1.));
#6903=DIRECTION('center_axis',(1.,0.,0.));
#6904=DIRECTION('ref_axis',(0.,0.,-1.));
#6905=DIRECTION('center_axis',(1.,0.,0.));
#6906=DIRECTION('ref_axis',(0.,0.,-1.));
#6907=DIRECTION('center_axis',(1.,5.78241158658936E-16,0.));
#6908=DIRECTION('ref_axis',(-5.78241158658936E-16,1.,0.));
#6909=DIRECTION('center_axis',(1.,0.,0.));
#6910=DIRECTION('ref_axis',(0.,0.,-1.));
#6911=DIRECTION('center_axis',(-1.,0.,0.));
#6912=DIRECTION('ref_axis',(0.,0.,1.));
#6913=DIRECTION('center_axis',(-1.,0.,0.));
#6914=DIRECTION('ref_axis',(0.,0.,1.));
#6915=DIRECTION('center_axis',(-1.,0.,0.));
#6916=DIRECTION('ref_axis',(0.,0.,1.));
#6917=DIRECTION('center_axis',(-1.,0.,0.));
#6918=DIRECTION('ref_axis',(0.,0.,1.));
#6919=DIRECTION('center_axis',(-1.,0.,0.));
#6920=DIRECTION('ref_axis',(0.,0.,1.));
#6921=DIRECTION('center_axis',(-1.,0.,0.));
#6922=DIRECTION('ref_axis',(0.,0.,1.));
#6923=DIRECTION('center_axis',(-1.,0.,0.));
#6924=DIRECTION('ref_axis',(0.,0.,1.));
#6925=DIRECTION('center_axis',(-1.,0.,0.));
#6926=DIRECTION('ref_axis',(0.,0.,1.));
#6927=DIRECTION('center_axis',(-1.,0.,0.));
#6928=DIRECTION('ref_axis',(0.,0.,1.));
#6929=DIRECTION('center_axis',(-1.,0.,0.));
#6930=DIRECTION('ref_axis',(0.,0.,1.));
#6931=DIRECTION('center_axis',(-1.,0.,0.));
#6932=DIRECTION('ref_axis',(0.,0.,1.));
#6933=DIRECTION('center_axis',(-1.,0.,0.));
#6934=DIRECTION('ref_axis',(0.,0.,1.));
#6935=DIRECTION('center_axis',(-1.,0.,0.));
#6936=DIRECTION('ref_axis',(0.,0.,1.));
#7531=CARTESIAN_POINT('',(0.,0.,0.));
#7532=CARTESIAN_POINT('Origin',(0.0232500000002624,0.0199999999999376,0.0120000000000001));
#7533=CARTESIAN_POINT('',(0.02175,0.00499999999993959,0.012));
#7534=CARTESIAN_POINT('',(0.02175,0.0199999999999396,0.0120000000000001));
#7535=CARTESIAN_POINT('',(0.02175,0.0104999999999688,0.0120000000000001));
#7536=CARTESIAN_POINT('',(0.0232500000002423,0.00499999999993758,0.012));
#7537=CARTESIAN_POINT('',(0.0232500000002423,0.00499999999993758,0.012));
#7538=CARTESIAN_POINT('',(0.0232500000002624,0.0199999999999376,0.0120000000000001));
#7539=CARTESIAN_POINT('',(0.02325,0.00999999999996881,0.0120000000000001));
#7540=CARTESIAN_POINT('',(0.0116250000001312,0.02,0.0120000000000001));
#7541=CARTESIAN_POINT('Origin',(0.0232500000002422,0.00499999999993754,
0.032));
#7542=CARTESIAN_POINT('',(0.02175,0.0199999999999396,0.0320000000000001));
#7543=CARTESIAN_POINT('',(0.02175,0.00499999999993952,0.032));
#7544=CARTESIAN_POINT('',(0.02175,0.00299999999996879,0.032));
#7545=CARTESIAN_POINT('',(0.0232500000002624,0.0199999999999376,0.0320000000000001));
#7546=CARTESIAN_POINT('',(0.0116250000001211,0.02,0.0320000000000001));
#7547=CARTESIAN_POINT('',(0.0232500000002422,0.00499999999993751,0.032));
#7548=CARTESIAN_POINT('',(0.02325,0.00249999999996874,0.032));
#7549=CARTESIAN_POINT('',(0.0232500000002422,0.00499999999993751,0.032));
#7550=CARTESIAN_POINT('Origin',(0.0232500000002423,0.00499999999993758,
0.012));
#7551=CARTESIAN_POINT('',(0.02175,0.00499999999993956,0.029));
#7552=CARTESIAN_POINT('',(0.02325,0.00499999999993759,0.00700000000000003));
#7553=CARTESIAN_POINT('Origin',(0.,0.02,0.002));
#7554=CARTESIAN_POINT('',(0.02325,0.02,0.));
#7555=CARTESIAN_POINT('',(0.02325,0.02,0.002));
#7556=CARTESIAN_POINT('',(-0.02325,0.02,0.));
#7557=CARTESIAN_POINT('',(0.,0.02,0.));
#7558=CARTESIAN_POINT('',(-0.02325,0.02,0.012));
#7559=CARTESIAN_POINT('',(-0.02325,0.02,0.002));
#7560=CARTESIAN_POINT('',(-0.02175,0.02,0.012));
#7561=CARTESIAN_POINT('',(-0.01325,0.02,0.012));
#7562=CARTESIAN_POINT('',(-0.02175,0.02,0.002));
#7563=CARTESIAN_POINT('',(-0.02175,0.02,0.046));
#7564=CARTESIAN_POINT('',(0.02175,0.02,0.002));
#7565=CARTESIAN_POINT('',(0.,0.02,0.002));
#7566=CARTESIAN_POINT('',(0.02175,0.02,0.046));
#7567=CARTESIAN_POINT('Origin',(0.,0.02,0.002));
#7568=CARTESIAN_POINT('',(0.02175,0.02,0.046));
#7569=CARTESIAN_POINT('',(0.02175,0.02,0.046));
#7570=CARTESIAN_POINT('',(-0.02175,0.02,0.046));
#7571=CARTESIAN_POINT('',(0.,0.02,0.046));
#7572=CARTESIAN_POINT('',(-0.02175,0.02,0.032));
#7573=CARTESIAN_POINT('',(-0.02175,0.02,0.046));
#7574=CARTESIAN_POINT('',(-0.02325,0.02,0.032));
#7575=CARTESIAN_POINT('',(-0.01325,0.02,0.032));
#7576=CARTESIAN_POINT('',(-0.02325,0.02,0.051));
#7577=CARTESIAN_POINT('',(-0.02325,0.02,0.002));
#7578=CARTESIAN_POINT('',(0.02325,0.02,0.051));
#7579=CARTESIAN_POINT('',(0.,0.02,0.051));
#7580=CARTESIAN_POINT('',(0.02325,0.02,0.002));
#7581=CARTESIAN_POINT('Origin',(0.02175,0.001,0.046));
#7582=CARTESIAN_POINT('',(0.02175,-0.018,0.002));
#7583=CARTESIAN_POINT('',(0.02175,0.001,0.002));
#7584=CARTESIAN_POINT('',(0.02175,-0.018,0.046));
#7585=CARTESIAN_POINT('',(0.02175,-0.018,0.046));
#7586=CARTESIAN_POINT('',(0.02175,0.001,0.046));
#7587=CARTESIAN_POINT('Origin',(0.0232500000002423,0.00500000000000003,
0.0560000000000001));
#7588=CARTESIAN_POINT('',(-0.02325,0.005,0.051));
#7589=CARTESIAN_POINT('',(-0.02325,0.00500000000006252,0.0560000000000001));
#7590=CARTESIAN_POINT('',(-0.02325,0.0050000000000625,0.0547500000000001));
#7591=CARTESIAN_POINT('',(0.0232500000002422,0.00500000000000004,0.0560000000000001));
#7592=CARTESIAN_POINT('',(1.24499124710741E-13,0.00500000000003127,0.0560000000000001));
#7593=CARTESIAN_POINT('',(0.02325,0.005,0.051));
#7594=CARTESIAN_POINT('',(0.0232500000002423,0.005,0.0510000000000001));
#7595=CARTESIAN_POINT('',(0.02325,0.005,0.051));
#7596=CARTESIAN_POINT('Origin',(-0.0232499999999731,0.0199999999998699,
0.0560000000000001));
#7597=CARTESIAN_POINT('',(-0.0232499999999731,0.0199999999998699,0.0560000000000001));
#7598=CARTESIAN_POINT('',(-0.0232499999999731,0.0199999999998699,0.0560000000000001));
#7599=CARTESIAN_POINT('',(0.0232500000000269,0.0199999999998074,0.0560000000000001));
#7600=CARTESIAN_POINT('',(0.0232500000000269,0.0199999999998074,0.0560000000000001));
#7601=CARTESIAN_POINT('',(0.0232500000000269,0.0199999999998074,0.0560000000000001));
#7602=CARTESIAN_POINT('Origin',(2.69118061169138E-14,0.0199999999998387,
0.0585000000000001));
#7603=CARTESIAN_POINT('',(-0.0232499999999731,0.0199999999998699,0.0610000000000001));
#7604=CARTESIAN_POINT('',(0.0232500000000269,0.0199999999998075,0.0610000000000001));
#7605=CARTESIAN_POINT('',(-0.0232499999999731,0.0199999999998699,0.0610000000000001));
#7606=CARTESIAN_POINT('',(0.0232500000000269,0.0199999999998075,0.0610000000000001));
#7607=CARTESIAN_POINT('',(-0.0232499999999731,0.0199999999998699,0.0560000000000001));
#7608=CARTESIAN_POINT('Origin',(0.,0.,0.046));
#7609=CARTESIAN_POINT('',(-0.02175,-0.018,0.046));
#7610=CARTESIAN_POINT('',(-0.02175,0.001,0.046));
#7611=CARTESIAN_POINT('',(6.93889390390723E-18,-0.018,0.046));
#7612=CARTESIAN_POINT('',(-0.01825,-0.0127,0.046));
#7613=CARTESIAN_POINT('',(-0.01825,-0.0175,0.046));
#7614=CARTESIAN_POINT('',(-0.01825,-0.01625,0.046));
#7615=CARTESIAN_POINT('',(-0.02125,-0.0127,0.046));
#7616=CARTESIAN_POINT('',(0.,-0.0127,0.046));
#7617=CARTESIAN_POINT('',(-0.02125,-0.0175,0.046));
#7618=CARTESIAN_POINT('',(-0.02125,-0.01625,0.046));
#7619=CARTESIAN_POINT('',(-0.01975,-0.0175,0.046));
#7620=CARTESIAN_POINT('',(0.00525,-0.0127,0.046));
#7621=CARTESIAN_POINT('',(0.00525,-0.0175,0.046));
#7622=CARTESIAN_POINT('',(0.00525,-0.01625,0.046));
#7623=CARTESIAN_POINT('',(0.00225,-0.0127,0.046));
#7624=CARTESIAN_POINT('',(7.3436627149685E-18,-0.0127,0.046));
#7625=CARTESIAN_POINT('',(0.00225,-0.0175,0.046));
#7626=CARTESIAN_POINT('',(0.00225,-0.01625,0.046));
#7627=CARTESIAN_POINT('',(0.00375,-0.0175,0.046));
#7628=CARTESIAN_POINT('',(0.01825,-0.0073,0.046));
#7629=CARTESIAN_POINT('',(0.02125,-0.0073,0.046));
#7630=CARTESIAN_POINT('',(0.02125,-0.0073,0.046));
#7631=CARTESIAN_POINT('',(0.02125,-0.0025,0.046));
#7632=CARTESIAN_POINT('',(0.02125,-0.00375,0.046));
#7633=CARTESIAN_POINT('',(0.01825,-0.0025,0.046));
#7634=CARTESIAN_POINT('',(0.01975,-0.0025,0.046));
#7635=CARTESIAN_POINT('',(0.01825,-0.00375,0.046));
#7636=CARTESIAN_POINT('',(-0.00525,-0.0073,0.046));
#7637=CARTESIAN_POINT('',(-0.00225,-0.0073,0.046));
#7638=CARTESIAN_POINT('',(-0.00225,-0.0073,0.046));
#7639=CARTESIAN_POINT('',(-0.00225,-0.0025,0.046));
#7640=CARTESIAN_POINT('',(-0.00225,-0.00375,0.046));
#7641=CARTESIAN_POINT('',(-0.00525,-0.0025,0.046));
#7642=CARTESIAN_POINT('',(-0.00375,-0.0025,0.046));
#7643=CARTESIAN_POINT('',(-0.00525,-0.00375,0.046));
#7644=CARTESIAN_POINT('',(0.00225,-0.0073,0.046));
#7645=CARTESIAN_POINT('',(0.00525,-0.0073,0.046));
#7646=CARTESIAN_POINT('',(0.00525,-0.0073,0.046));
#7647=CARTESIAN_POINT('',(0.00525,-0.0025,0.046));
#7648=CARTESIAN_POINT('',(0.00525,-0.00375,0.046));
#7649=CARTESIAN_POINT('',(0.00225,-0.0025,0.046));
#7650=CARTESIAN_POINT('',(0.00375,-0.0025,0.046));
#7651=CARTESIAN_POINT('',(0.00225,-0.00375,0.046));
#7652=CARTESIAN_POINT('',(0.02125,-0.0127,0.046));
#7653=CARTESIAN_POINT('',(0.02125,-0.0175,0.046));
#7654=CARTESIAN_POINT('',(0.02125,-0.01625,0.046));
#7655=CARTESIAN_POINT('',(0.01825,-0.0127,0.046));
#7656=CARTESIAN_POINT('',(0.,-0.0127,0.046));
#7657=CARTESIAN_POINT('',(0.01825,-0.0175,0.046));
#7658=CARTESIAN_POINT('',(0.01825,-0.01625,0.046));
#7659=CARTESIAN_POINT('',(0.01975,-0.0175,0.046));
#7660=CARTESIAN_POINT('',(-0.00225,-0.0127,0.046));
#7661=CARTESIAN_POINT('',(-0.00525,-0.0127,0.046));
#7662=CARTESIAN_POINT('',(-0.00525,-0.0127,0.046));
#7663=CARTESIAN_POINT('',(-0.00525,-0.0175,0.046));
#7664=CARTESIAN_POINT('',(-0.00525,-0.01625,0.046));
#7665=CARTESIAN_POINT('',(-0.00225,-0.0175,0.046));
#7666=CARTESIAN_POINT('',(-0.00375,-0.0175,0.046));
#7667=CARTESIAN_POINT('',(-0.00225,-0.01625,0.046));
#7668=CARTESIAN_POINT('',(-0.02125,-0.0073,0.046));
#7669=CARTESIAN_POINT('',(-0.01825,-0.0073,0.046));
#7670=CARTESIAN_POINT('',(-0.01825,-0.0073,0.046));
#7671=CARTESIAN_POINT('',(-0.01825,-0.0025,0.046));
#7672=CARTESIAN_POINT('',(-0.01825,-0.00375,0.046));
#7673=CARTESIAN_POINT('',(-0.02125,-0.0025,0.046));
#7674=CARTESIAN_POINT('',(-0.01975,-0.0025,0.046));
#7675=CARTESIAN_POINT('',(-0.02125,-0.00375,0.046));
#7676=CARTESIAN_POINT('Origin',(0.01825,-0.01625,0.061));
#7677=CARTESIAN_POINT('',(0.01825,-0.017211102550928,0.061));
#7678=CARTESIAN_POINT('',(0.01825,-0.0175,0.0598288205727445));
#7679=CARTESIAN_POINT('Origin',(0.01825,-0.01,0.0586));
#7680=CARTESIAN_POINT('',(0.01825,-0.0175,0.061));
#7681=CARTESIAN_POINT('',(0.01825,-0.01625,0.061));
#7682=CARTESIAN_POINT('',(0.01825,-0.0175,0.061));
#7683=CARTESIAN_POINT('Origin',(0.02125,-0.01625,0.061));
#7684=CARTESIAN_POINT('',(0.02125,-0.017211102550928,0.061));
#7685=CARTESIAN_POINT('',(0.02125,-0.0175,0.061));
#7686=CARTESIAN_POINT('',(0.02125,-0.01625,0.061));
#7687=CARTESIAN_POINT('',(0.02125,-0.0175,0.0598288205727445));
#7688=CARTESIAN_POINT('Origin',(0.02125,-0.01,0.0586));
#7689=CARTESIAN_POINT('',(0.02125,-0.0175,0.061));
#7690=CARTESIAN_POINT('Origin',(0.00225,-0.01625,0.061));
#7691=CARTESIAN_POINT('',(0.00225,-0.017211102550928,0.061));
#7692=CARTESIAN_POINT('',(0.00225,-0.0175,0.0598288205727445));
#7693=CARTESIAN_POINT('Origin',(0.00225,-0.01,0.0586));
#7694=CARTESIAN_POINT('',(0.00225,-0.0175,0.061));
#7695=CARTESIAN_POINT('',(0.00225,-0.01625,0.061));
#7696=CARTESIAN_POINT('',(0.00225,-0.0175,0.061));
#7697=CARTESIAN_POINT('Origin',(0.00525,-0.01625,0.061));
#7698=CARTESIAN_POINT('',(0.00525,-0.017211102550928,0.061));
#7699=CARTESIAN_POINT('',(0.00525,-0.0175,0.061));
#7700=CARTESIAN_POINT('',(0.00525,-0.01625,0.061));
#7701=CARTESIAN_POINT('',(0.00525,-0.0175,0.0598288205727445));
#7702=CARTESIAN_POINT('Origin',(0.00525,-0.01,0.0586));
#7703=CARTESIAN_POINT('',(0.00525,-0.0175,0.061));
#7704=CARTESIAN_POINT('Origin',(0.00225,-0.00375,0.061));
#7705=CARTESIAN_POINT('',(0.00225,-0.0025,0.0598288205727444));
#7706=CARTESIAN_POINT('',(0.00225,-0.00278889744907202,0.061));
#7707=CARTESIAN_POINT('Origin',(0.00225,-0.01,0.0586));
#7708=CARTESIAN_POINT('',(0.00225,-0.0025,0.061));
#7709=CARTESIAN_POINT('',(0.00225,-0.0025,0.061));
#7710=CARTESIAN_POINT('',(0.00225,-0.00375,0.061));
#7711=CARTESIAN_POINT('Origin',(-0.00225,-0.01625,0.061));
#7712=CARTESIAN_POINT('',(-0.00225,-0.0175,0.0598288205727445));
#7713=CARTESIAN_POINT('',(-0.00225,-0.017211102550928,0.061));
#7714=CARTESIAN_POINT('Origin',(-0.00225,-0.01,0.0586));
#7715=CARTESIAN_POINT('',(-0.00225,-0.0175,0.061));
#7716=CARTESIAN_POINT('',(-0.00225,-0.0175,0.061));
#7717=CARTESIAN_POINT('',(-0.00225,-0.01625,0.061));
#7718=CARTESIAN_POINT('Origin',(-0.00375,-0.0175,0.061));
#7719=CARTESIAN_POINT('',(-0.00525,-0.0175,0.0598288205727445));
#7720=CARTESIAN_POINT('',(0.02675,-0.0175,0.0598288205727445));
#7721=CARTESIAN_POINT('',(-0.00525,-0.0175,0.061));
#7722=CARTESIAN_POINT('',(-0.00525,-0.0175,0.061));
#7723=CARTESIAN_POINT('',(-0.00375,-0.0175,0.061));
#7724=CARTESIAN_POINT('Origin',(-0.00225,-0.00375,0.061));
#7725=CARTESIAN_POINT('',(-0.00225,-0.0025,0.061));
#7726=CARTESIAN_POINT('',(-0.00225,-0.0025,0.0598288205727444));
#7727=CARTESIAN_POINT('',(-0.00225,-0.0025,0.061));
#7728=CARTESIAN_POINT('',(-0.00225,-0.00278889744907202,0.061));
#7729=CARTESIAN_POINT('Origin',(-0.00225,-0.01,0.0586));
#7730=CARTESIAN_POINT('',(-0.00225,-0.00375,0.061));
#7731=CARTESIAN_POINT('Origin',(-0.02125,-0.01625,0.061));
#7732=CARTESIAN_POINT('',(-0.02125,-0.017211102550928,0.061));
#7733=CARTESIAN_POINT('',(-0.02125,-0.0175,0.0598288205727445));
#7734=CARTESIAN_POINT('Origin',(-0.02125,-0.01,0.0586));
#7735=CARTESIAN_POINT('',(-0.02125,-0.0175,0.061));
#7736=CARTESIAN_POINT('',(-0.02125,-0.01625,0.061));
#7737=CARTESIAN_POINT('',(-0.02125,-0.0175,0.061));
#7738=CARTESIAN_POINT('Origin',(-0.01825,-0.01625,0.061));
#7739=CARTESIAN_POINT('',(-0.01825,-0.017211102550928,0.061));
#7740=CARTESIAN_POINT('',(-0.01825,-0.0175,0.061));
#7741=CARTESIAN_POINT('',(-0.01825,-0.01625,0.061));
#7742=CARTESIAN_POINT('',(-0.01825,-0.0175,0.0598288205727445));
#7743=CARTESIAN_POINT('Origin',(-0.01825,-0.01,0.0586));
#7744=CARTESIAN_POINT('',(-0.01825,-0.0175,0.061));
#7745=CARTESIAN_POINT('Origin',(-3.46944695195361E-18,0.,0.061));
#7746=CARTESIAN_POINT('',(0.02325,-0.017211102550928,0.061));
#7747=CARTESIAN_POINT('',(0.02325,-0.02,0.061));
#7748=CARTESIAN_POINT('',(0.02325,3.46944695195361E-18,0.061));
#7749=CARTESIAN_POINT('',(0.02675,-0.017211102550928,0.061));
#7750=CARTESIAN_POINT('',(0.01975,-0.0175,0.061));
#7751=CARTESIAN_POINT('',(0.02675,-0.017211102550928,0.061));
#7752=CARTESIAN_POINT('',(0.00375,-0.0175,0.061));
#7753=CARTESIAN_POINT('',(0.02675,-0.017211102550928,0.061));
#7754=CARTESIAN_POINT('',(-0.00525,-0.017211102550928,0.061));
#7755=CARTESIAN_POINT('',(-0.00525,-0.01625,0.061));
#7756=CARTESIAN_POINT('',(0.02675,-0.017211102550928,0.061));
#7757=CARTESIAN_POINT('',(-0.01975,-0.0175,0.061));
#7758=CARTESIAN_POINT('',(-0.02325,-0.017211102550928,0.061));
#7759=CARTESIAN_POINT('',(0.02675,-0.017211102550928,0.061));
#7760=CARTESIAN_POINT('',(-0.02325,-0.02,0.061));
#7761=CARTESIAN_POINT('',(-0.02325,-3.46944695195361E-18,0.061));
#7762=CARTESIAN_POINT('',(0.,-0.02,0.061));
#7763=CARTESIAN_POINT('Origin',(0.,0.,0.051));
#7764=CARTESIAN_POINT('',(-0.02325,-3.46944695195361E-18,0.051));
#7765=CARTESIAN_POINT('',(0.02325,3.46944695195361E-18,0.051));
#7766=CARTESIAN_POINT('Origin',(0.,0.,0.002));
#7767=CARTESIAN_POINT('',(-0.02175,-0.018,0.002));
#7768=CARTESIAN_POINT('',(-0.02175,0.001,0.002));
#7769=CARTESIAN_POINT('',(6.93889390390723E-18,-0.018,0.002));
#7770=CARTESIAN_POINT('',(-0.02125,-0.0127,0.002));
#7771=CARTESIAN_POINT('',(-0.02125,-0.0175,0.002));
#7772=CARTESIAN_POINT('',(-0.02125,0.,0.002));
#7773=CARTESIAN_POINT('',(-0.01825,-0.0127,0.002));
#7774=CARTESIAN_POINT('',(0.,-0.0127,0.002));
#7775=CARTESIAN_POINT('',(-0.01825,-0.0175,0.002));
#7776=CARTESIAN_POINT('',(-0.01825,0.,0.002));
#7777=CARTESIAN_POINT('',(0.,-0.0175,0.002));
#7778=CARTESIAN_POINT('',(-0.01825,-0.0073,0.002));
#7779=CARTESIAN_POINT('',(-0.02125,-0.0073,0.002));
#7780=CARTESIAN_POINT('',(-0.02125,-0.0073,0.002));
#7781=CARTESIAN_POINT('',(-0.02125,-0.0025,0.002));
#7782=CARTESIAN_POINT('',(-0.02125,0.,0.002));
#7783=CARTESIAN_POINT('',(-0.01825,-0.0025,0.002));
#7784=CARTESIAN_POINT('',(0.,-0.0025,0.002));
#7785=CARTESIAN_POINT('',(-0.01825,0.,0.002));
#7786=CARTESIAN_POINT('',(-0.00225,-0.0073,0.002));
#7787=CARTESIAN_POINT('',(-0.00225,-0.0025,0.002));
#7788=CARTESIAN_POINT('',(-0.00225,3.90312782094781E-19,0.002));
#7789=CARTESIAN_POINT('',(-0.00525,-0.0073,0.002));
#7790=CARTESIAN_POINT('',(-2.11058022910511E-18,-0.0073,0.002));
#7791=CARTESIAN_POINT('',(-0.00525,-0.0025,0.002));
#7792=CARTESIAN_POINT('',(-0.00525,0.,0.002));
#7793=CARTESIAN_POINT('',(-3.61400724161836E-19,-0.0025,0.002));
#7794=CARTESIAN_POINT('',(0.00525,-0.0073,0.002));
#7795=CARTESIAN_POINT('',(0.00225,-0.0073,0.002));
#7796=CARTESIAN_POINT('',(0.00225,-0.0073,0.002));
#7797=CARTESIAN_POINT('',(0.00225,-0.0025,0.002));
#7798=CARTESIAN_POINT('',(0.00225,-3.90312782094781E-19,0.002));
#7799=CARTESIAN_POINT('',(0.00525,-0.0025,0.002));
#7800=CARTESIAN_POINT('',(-7.2280144832367E-19,-0.0025,0.002));
#7801=CARTESIAN_POINT('',(0.00525,0.,0.002));
#7802=CARTESIAN_POINT('',(0.02125,-0.0073,0.002));
#7803=CARTESIAN_POINT('',(0.01825,-0.0073,0.002));
#7804=CARTESIAN_POINT('',(0.01825,-0.0073,0.002));
#7805=CARTESIAN_POINT('',(0.01825,-0.0025,0.002));
#7806=CARTESIAN_POINT('',(0.01825,0.,0.002));
#7807=CARTESIAN_POINT('',(0.02125,-0.0025,0.002));
#7808=CARTESIAN_POINT('',(0.,-0.0025,0.002));
#7809=CARTESIAN_POINT('',(0.02125,0.,0.002));
#7810=CARTESIAN_POINT('',(0.01825,-0.0127,0.002));
#7811=CARTESIAN_POINT('',(0.01825,-0.0175,0.002));
#7812=CARTESIAN_POINT('',(0.01825,0.,0.002));
#7813=CARTESIAN_POINT('',(0.02125,-0.0127,0.002));
#7814=CARTESIAN_POINT('',(0.,-0.0127,0.002));
#7815=CARTESIAN_POINT('',(0.02125,-0.0175,0.002));
#7816=CARTESIAN_POINT('',(0.02125,0.,0.002));
#7817=CARTESIAN_POINT('',(0.,-0.0175,0.002));
#7818=CARTESIAN_POINT('',(0.00225,-0.0127,0.002));
#7819=CARTESIAN_POINT('',(0.00225,-0.0175,0.002));
#7820=CARTESIAN_POINT('',(0.00225,-3.90312782094782E-19,0.002));
#7821=CARTESIAN_POINT('',(0.00525,-0.0127,0.002));
#7822=CARTESIAN_POINT('',(0.,-0.0127,0.002));
#7823=CARTESIAN_POINT('',(0.00525,-0.0175,0.002));
#7824=CARTESIAN_POINT('',(0.00525,0.,0.002));
#7825=CARTESIAN_POINT('',(0.,-0.0175,0.002));
#7826=CARTESIAN_POINT('',(-0.00525,-0.0127,0.002));
#7827=CARTESIAN_POINT('',(-0.00525,-0.0175,0.002));
#7828=CARTESIAN_POINT('',(-0.00525,0.,0.002));
#7829=CARTESIAN_POINT('',(-0.00225,-0.0127,0.002));
#7830=CARTESIAN_POINT('',(-7.34366271496849E-18,-0.0127,0.002));
#7831=CARTESIAN_POINT('',(-0.00225,-0.0175,0.002));
#7832=CARTESIAN_POINT('',(-0.00225,3.90312782094781E-19,0.002));
#7833=CARTESIAN_POINT('',(0.,-0.0175,0.002));
#7834=CARTESIAN_POINT('Origin',(0.01825,-0.00375,-0.01));
#7835=CARTESIAN_POINT('',(0.01825,-0.00278889744907202,-0.01));
#7836=CARTESIAN_POINT('',(0.01825,-0.0025,-0.00882882057274445));
#7837=CARTESIAN_POINT('Origin',(0.01825,-0.01,-0.0076));
#7838=CARTESIAN_POINT('',(0.01825,-0.0025,-0.01));
#7839=CARTESIAN_POINT('',(0.01825,-0.00375,-0.01));
#7840=CARTESIAN_POINT('',(0.01825,-0.0025,-0.01));
#7841=CARTESIAN_POINT('Origin',(0.02125,-0.00375,-0.01));
#7842=CARTESIAN_POINT('',(0.02125,-0.00278889744907202,-0.01));
#7843=CARTESIAN_POINT('',(0.02125,-0.0025,-0.01));
#7844=CARTESIAN_POINT('',(0.02125,-0.00375,-0.01));
#7845=CARTESIAN_POINT('',(0.02125,-0.0025,-0.00882882057274445));
#7846=CARTESIAN_POINT('Origin',(0.02125,-0.01,-0.0076));
#7847=CARTESIAN_POINT('',(0.02125,-0.0025,-0.01));
#7848=CARTESIAN_POINT('Origin',(0.00525,-0.00375,-0.01));
#7849=CARTESIAN_POINT('',(0.00525,-0.00278889744907202,-0.01));
#7850=CARTESIAN_POINT('',(0.00525,-0.0025,-0.01));
#7851=CARTESIAN_POINT('',(0.00525,-0.00375,-0.01));
#7852=CARTESIAN_POINT('',(0.00525,-0.0025,-0.00882882057274439));
#7853=CARTESIAN_POINT('Origin',(0.00525,-0.01,-0.0076));
#7854=CARTESIAN_POINT('',(0.00525,-0.0025,-0.01));
#7855=CARTESIAN_POINT('Origin',(0.01975,-0.0175,-0.01));
#7856=CARTESIAN_POINT('',(0.01825,-0.0175,-0.01));
#7857=CARTESIAN_POINT('',(0.01825,-0.0175,-0.00882882057274447));
#7858=CARTESIAN_POINT('',(0.01825,-0.0175,-0.01));
#7859=CARTESIAN_POINT('',(0.02125,-0.0175,-0.00882882057274447));
#7860=CARTESIAN_POINT('',(-0.02675,-0.0175,-0.00882882057274447));
#7861=CARTESIAN_POINT('',(0.02125,-0.0175,-0.01));
#7862=CARTESIAN_POINT('',(0.02125,-0.0175,-0.01));
#7863=CARTESIAN_POINT('',(0.01975,-0.0175,-0.01));
#7864=CARTESIAN_POINT('Origin',(0.00375,-0.0175,-0.01));
#7865=CARTESIAN_POINT('',(0.00225,-0.0175,-0.01));
#7866=CARTESIAN_POINT('',(0.00225,-0.0175,-0.00882882057274447));
#7867=CARTESIAN_POINT('',(0.00225,-0.0175,-0.01));
#7868=CARTESIAN_POINT('',(0.00525,-0.0175,-0.00882882057274447));
#7869=CARTESIAN_POINT('',(-0.02675,-0.0175,-0.00882882057274447));
#7870=CARTESIAN_POINT('',(0.00525,-0.0175,-0.01));
#7871=CARTESIAN_POINT('',(0.00525,-0.0175,-0.01));
#7872=CARTESIAN_POINT('',(0.00375,-0.0175,-0.01));
#7873=CARTESIAN_POINT('Origin',(-0.00375,-0.0175,-0.01));
#7874=CARTESIAN_POINT('',(-0.00525,-0.0175,-0.01));
#7875=CARTESIAN_POINT('',(-0.00525,-0.0175,-0.00882882057274447));
#7876=CARTESIAN_POINT('',(-0.00525,-0.0175,-0.01));
#7877=CARTESIAN_POINT('',(-0.00225,-0.0175,-0.00882882057274447));
#7878=CARTESIAN_POINT('',(-0.02675,-0.0175,-0.00882882057274447));
#7879=CARTESIAN_POINT('',(-0.00225,-0.0175,-0.01));
#7880=CARTESIAN_POINT('',(-0.00225,-0.0175,-0.01));
#7881=CARTESIAN_POINT('',(-0.00375,-0.0175,-0.01));
#7882=CARTESIAN_POINT('Origin',(-0.02125,-0.00375,-0.01));
#7883=CARTESIAN_POINT('',(-0.02125,-0.00278889744907202,-0.01));
#7884=CARTESIAN_POINT('',(-0.02125,-0.0025,-0.00882882057274445));
#7885=CARTESIAN_POINT('Origin',(-0.02125,-0.01,-0.0076));
#7886=CARTESIAN_POINT('',(-0.02125,-0.0025,-0.01));
#7887=CARTESIAN_POINT('',(-0.02125,-0.00375,-0.01));
#7888=CARTESIAN_POINT('',(-0.02125,-0.0025,-0.01));
#7889=CARTESIAN_POINT('Origin',(-0.01825,-0.00375,-0.01));
#7890=CARTESIAN_POINT('',(-0.01825,-0.00278889744907202,-0.01));
#7891=CARTESIAN_POINT('',(-0.01825,-0.0025,-0.01));
#7892=CARTESIAN_POINT('',(-0.01825,-0.00375,-0.01));
#7893=CARTESIAN_POINT('',(-0.01825,-0.0025,-0.00882882057274445));
#7894=CARTESIAN_POINT('Origin',(-0.01825,-0.01,-0.0076));
#7895=CARTESIAN_POINT('',(-0.01825,-0.0025,-0.01));
#7896=CARTESIAN_POINT('Origin',(-0.01975,-0.0175,-0.01));
#7897=CARTESIAN_POINT('',(-0.02125,-0.0175,-0.01));
#7898=CARTESIAN_POINT('',(-0.02125,-0.0175,-0.00882882057274447));
#7899=CARTESIAN_POINT('',(-0.02125,-0.0175,-0.01));
#7900=CARTESIAN_POINT('',(-0.01825,-0.0175,-0.00882882057274447));
#7901=CARTESIAN_POINT('',(-0.02675,-0.0175,-0.00882882057274447));
#7902=CARTESIAN_POINT('',(-0.01825,-0.0175,-0.01));
#7903=CARTESIAN_POINT('',(-0.01825,-0.0175,-0.01));
#7904=CARTESIAN_POINT('',(-0.01975,-0.0175,-0.01));
#7905=CARTESIAN_POINT('Origin',(0.01975,-0.0025,-0.01));
#7906=CARTESIAN_POINT('',(-0.02675,-0.0025,-0.00882882057274445));
#7907=CARTESIAN_POINT('',(0.01975,-0.0025,-0.01));
#7908=CARTESIAN_POINT('Origin',(0.00375,-0.0025,-0.01));
#7909=CARTESIAN_POINT('',(0.00225,-0.0025,-0.00882882057274439));
#7910=CARTESIAN_POINT('',(-0.02675,-0.0025,-0.00882882057274439));
#7911=CARTESIAN_POINT('',(0.00225,-0.0025,-0.01));
#7912=CARTESIAN_POINT('',(0.00225,-0.0025,-0.01));
#7913=CARTESIAN_POINT('',(0.00375,-0.0025,-0.01));
#7914=CARTESIAN_POINT('Origin',(-0.01975,-0.0025,-0.01));
#7915=CARTESIAN_POINT('',(-0.02675,-0.0025,-0.00882882057274445));
#7916=CARTESIAN_POINT('',(-0.01975,-0.0025,-0.01));
#7917=CARTESIAN_POINT('Origin',(0.,0.,-0.01));
#7918=CARTESIAN_POINT('',(-0.02325,-0.017211102550928,-0.01));
#7919=CARTESIAN_POINT('',(-0.02325,-0.02,-0.01));
#7920=CARTESIAN_POINT('',(-0.02325,-3.46944695195361E-18,-0.01));
#7921=CARTESIAN_POINT('',(-0.02125,-0.017211102550928,-0.01));
#7922=CARTESIAN_POINT('',(-0.02675,-0.017211102550928,-0.01));
#7923=CARTESIAN_POINT('',(-0.02125,-0.01625,-0.01));
#7924=CARTESIAN_POINT('',(-0.01825,-0.017211102550928,-0.01));
#7925=CARTESIAN_POINT('',(-0.01825,-0.01625,-0.01));
#7926=CARTESIAN_POINT('',(-0.00525,-0.017211102550928,-0.01));
#7927=CARTESIAN_POINT('',(-0.02675,-0.017211102550928,-0.01));
#7928=CARTESIAN_POINT('',(-0.00525,-0.01625,-0.01));
#7929=CARTESIAN_POINT('',(-0.00225,-0.017211102550928,-0.01));
#7930=CARTESIAN_POINT('',(-0.00225,-0.01625,-0.01));
#7931=CARTESIAN_POINT('',(0.00225,-0.017211102550928,-0.01));
#7932=CARTESIAN_POINT('',(-0.02675,-0.017211102550928,-0.01));
#7933=CARTESIAN_POINT('',(0.00225,-0.01625,-0.01));
#7934=CARTESIAN_POINT('',(0.00525,-0.017211102550928,-0.01));
#7935=CARTESIAN_POINT('',(0.00525,-0.01625,-0.01));
#7936=CARTESIAN_POINT('',(0.01825,-0.017211102550928,-0.01));
#7937=CARTESIAN_POINT('',(-0.02675,-0.017211102550928,-0.01));
#7938=CARTESIAN_POINT('',(0.01825,-0.01625,-0.01));
#7939=CARTESIAN_POINT('',(0.02125,-0.017211102550928,-0.01));
#7940=CARTESIAN_POINT('',(0.02125,-0.01625,-0.01));
#7941=CARTESIAN_POINT('',(0.02325,-0.017211102550928,-0.01));
#7942=CARTESIAN_POINT('',(-0.02675,-0.017211102550928,-0.01));
#7943=CARTESIAN_POINT('',(0.02325,-0.02,-0.01));
#7944=CARTESIAN_POINT('',(0.02325,3.46944695195361E-18,-0.01));
#7945=CARTESIAN_POINT('',(0.,-0.02,-0.01));
#7946=CARTESIAN_POINT('Origin',(0.,0.,0.));
#7947=CARTESIAN_POINT('',(0.02325,0.005,0.));
#7948=CARTESIAN_POINT('',(0.02325,3.46944695195361E-18,0.));
#7949=CARTESIAN_POINT('',(-0.02325,0.005,0.));
#7950=CARTESIAN_POINT('',(-0.02325,0.005,0.));
#7951=CARTESIAN_POINT('',(-0.02325,-3.46944695195361E-18,0.));
#7952=CARTESIAN_POINT('Origin',(-0.02175,0.001,0.046));
#7953=CARTESIAN_POINT('',(-0.02175,0.005,0.032));
#7954=CARTESIAN_POINT('',(-0.02175,0.005,0.012));
#7955=CARTESIAN_POINT('',(-0.02175,0.005,0.046));
#7956=CARTESIAN_POINT('',(-0.02175,0.001,0.032));
#7957=CARTESIAN_POINT('',(-0.02175,-0.018,0.046));
#7958=CARTESIAN_POINT('',(-0.02175,0.001,0.012));
#7959=CARTESIAN_POINT('Origin',(-0.02325,-3.46944695195361E-18,0.002));
#7960=CARTESIAN_POINT('',(-0.02325,-0.00278889744907202,0.061));
#7961=CARTESIAN_POINT('Origin',(-0.02325,-0.01,0.0586));
#7962=CARTESIAN_POINT('',(-0.02325,-3.46944695195361E-18,0.061));
#7963=CARTESIAN_POINT('',(-0.02325,0.005,0.032));
#7964=CARTESIAN_POINT('',(-0.02325,0.0125,0.032));
#7965=CARTESIAN_POINT('',(-0.02325,0.005,0.012));
#7966=CARTESIAN_POINT('',(-0.02325,0.005,0.022));
#7967=CARTESIAN_POINT('',(-0.02325,0.0125,0.012));
#7968=CARTESIAN_POINT('',(-0.02325,-3.46944695195361E-18,-0.005));
#7969=CARTESIAN_POINT('Origin',(-0.02325,0.005,-0.005));
#7970=CARTESIAN_POINT('',(-0.02325,-3.46944695195361E-18,-0.01));
#7971=CARTESIAN_POINT('',(-0.02325,-3.46944695195361E-18,-0.01));
#7972=CARTESIAN_POINT('',(-0.02325,-0.00278889744907202,-0.01));
#7973=CARTESIAN_POINT('',(-0.02325,-3.46944695195361E-18,-0.01));
#7974=CARTESIAN_POINT('Origin',(-0.02325,-0.01,-0.0076));
#7975=CARTESIAN_POINT('',(-0.02325,-0.02,0.002));
#7976=CARTESIAN_POINT('Origin',(0.,-0.02,0.002));
#7977=CARTESIAN_POINT('',(0.02325,-0.02,0.002));
#7978=CARTESIAN_POINT('',(0.0155,-0.02,0.00888));
#7979=CARTESIAN_POINT('Origin',(0.0155,-0.02,0.00765));
#7980=CARTESIAN_POINT('',(-0.0155,-0.02,0.00888));
#7981=CARTESIAN_POINT('Origin',(-0.0155,-0.02,0.00765));
#7982=CARTESIAN_POINT('',(-0.0155,-0.02,0.03988));
#7983=CARTESIAN_POINT('Origin',(-0.0155,-0.02,0.03865));
#7984=CARTESIAN_POINT('',(0.0155,-0.02,0.03988));
#7985=CARTESIAN_POINT('Origin',(0.0155,-0.02,0.03865));
#7986=CARTESIAN_POINT('',(-1.53080849893419E-18,-0.02,0.03565));
#7987=CARTESIAN_POINT('Origin',(0.,-0.02,0.02315));
#7988=CARTESIAN_POINT('Origin',(0.02325,3.46944695195361E-18,0.002));
#7989=CARTESIAN_POINT('',(0.02325,-0.00278889744907202,0.061));
#7990=CARTESIAN_POINT('',(0.02325,3.46944695195361E-18,0.061));
#7991=CARTESIAN_POINT('Origin',(0.02325,-0.01,0.0586));
#7992=CARTESIAN_POINT('',(0.02325,-0.00278889744907202,-0.01));
#7993=CARTESIAN_POINT('Origin',(0.02325,-0.01,-0.0076));
#7994=CARTESIAN_POINT('',(0.02325,-3.46944695195361E-18,-0.01));
#7995=CARTESIAN_POINT('',(0.02325,3.46944695195361E-18,-0.01));
#7996=CARTESIAN_POINT('',(0.02325,-3.46944695195361E-18,-0.005));
#7997=CARTESIAN_POINT('',(0.02325,-3.46944695195361E-18,-0.01));
#7998=CARTESIAN_POINT('Origin',(0.02325,0.005,-0.005));
#7999=CARTESIAN_POINT('Origin',(6.93889390390723E-18,-0.018,0.046));
#8000=CARTESIAN_POINT('',(0.0155,-0.018,0.00888));
#8001=CARTESIAN_POINT('Origin',(0.0155,-0.018,0.00765));
#8002=CARTESIAN_POINT('',(-0.0155,-0.018,0.00888));
#8003=CARTESIAN_POINT('Origin',(-0.0155,-0.018,0.00765));
#8004=CARTESIAN_POINT('',(-0.0155,-0.018,0.03988));
#8005=CARTESIAN_POINT('Origin',(-0.0155,-0.018,0.03865));
#8006=CARTESIAN_POINT('',(0.0155,-0.018,0.03988));
#8007=CARTESIAN_POINT('Origin',(0.0155,-0.018,0.03865));
#8008=CARTESIAN_POINT('',(0.,-0.018,0.03565));
#8009=CARTESIAN_POINT('Origin',(0.,-0.018,0.02315));
#8010=CARTESIAN_POINT('Origin',(-0.01325,0.0125,0.032));
#8011=CARTESIAN_POINT('',(-0.01325,0.005,0.032));
#8012=CARTESIAN_POINT('Origin',(-0.01325,0.0125,0.012));
#8013=CARTESIAN_POINT('',(-0.01325,0.005,0.012));
#8014=CARTESIAN_POINT('Origin',(-0.01325,0.005,0.022));
#8015=CARTESIAN_POINT('Origin',(0.,-0.015,0.02315));
#8016=CARTESIAN_POINT('',(-1.53080849893419E-18,-0.015,0.03565));
#8017=CARTESIAN_POINT('Origin',(0.0155,-0.015,0.03865));
#8018=CARTESIAN_POINT('',(0.0155,-0.015,0.03988));
#8019=CARTESIAN_POINT('Origin',(-0.0155,-0.015,0.03865));
#8020=CARTESIAN_POINT('',(-0.0155,-0.015,0.03988));
#8021=CARTESIAN_POINT('Origin',(-0.0155,-0.015,0.00765));
#8022=CARTESIAN_POINT('',(-0.0155,-0.015,0.00888));
#8023=CARTESIAN_POINT('Origin',(0.0155,-0.015,0.00765));
#8024=CARTESIAN_POINT('',(0.0155,-0.015,0.00888));
#8025=CARTESIAN_POINT('Origin',(0.,-2.60208521396521E-18,-0.01));
#8026=CARTESIAN_POINT('',(0.02325,-2.60208521396521E-18,-0.005));
#8027=CARTESIAN_POINT('',(0.,-2.60208521396521E-18,-0.01));
#8028=CARTESIAN_POINT('Origin',(0.00225,-0.00375,-0.01));
#8029=CARTESIAN_POINT('',(0.00225,-0.00278889744907202,-0.01));
#8030=CARTESIAN_POINT('Origin',(0.00225,-0.01,-0.0076));
#8031=CARTESIAN_POINT('',(0.00225,-0.00375,-0.01));
#8032=CARTESIAN_POINT('Origin',(0.01825,-0.01625,-0.01));
#8033=CARTESIAN_POINT('Origin',(0.01825,-0.01,-0.0076));
#8034=CARTESIAN_POINT('Origin',(0.02125,-0.01625,-0.01));
#8035=CARTESIAN_POINT('Origin',(0.02125,-0.01,-0.0076));
#8036=CARTESIAN_POINT('Origin',(0.00225,-0.01625,-0.01));
#8037=CARTESIAN_POINT('Origin',(0.00225,-0.01,-0.0076));
#8038=CARTESIAN_POINT('Origin',(0.00525,-0.01625,-0.01));
#8039=CARTESIAN_POINT('Origin',(0.00525,-0.01,-0.0076));
#8040=CARTESIAN_POINT('Origin',(-0.00225,-0.00375,-0.01));
#8041=CARTESIAN_POINT('',(-0.00225,-0.0025,-0.00882882057274444));
#8042=CARTESIAN_POINT('',(-0.00225,-0.00278889744907202,-0.01));
#8043=CARTESIAN_POINT('Origin',(-0.00225,-0.01,-0.0076));
#8044=CARTESIAN_POINT('',(-0.00225,-0.0025,-0.01));
#8045=CARTESIAN_POINT('',(-0.00225,-0.0025,-0.01));
#8046=CARTESIAN_POINT('',(-0.00225,-0.00375,-0.01));
#8047=CARTESIAN_POINT('Origin',(-0.00375,-0.0025,-0.01));
#8048=CARTESIAN_POINT('',(-0.00525,-0.0025,-0.00882882057274445));
#8049=CARTESIAN_POINT('',(-0.02675,-0.0025,-0.00882882057274444));
#8050=CARTESIAN_POINT('',(-0.00525,-0.0025,-0.01));
#8051=CARTESIAN_POINT('',(-0.00525,-0.0025,-0.01));
#8052=CARTESIAN_POINT('',(-0.00375,-0.0025,-0.01));
#8053=CARTESIAN_POINT('Origin',(-0.00525,-0.00375,-0.01));
#8054=CARTESIAN_POINT('',(-0.00525,-0.00278889744907202,-0.01));
#8055=CARTESIAN_POINT('Origin',(-0.00525,-0.01,-0.0076));
#8056=CARTESIAN_POINT('',(-0.00525,-0.00375,-0.01));
#8057=CARTESIAN_POINT('Origin',(-0.00525,-0.01625,-0.01));
#8058=CARTESIAN_POINT('Origin',(-0.00525,-0.01,-0.0076));
#8059=CARTESIAN_POINT('Origin',(-0.00225,-0.01625,-0.01));
#8060=CARTESIAN_POINT('Origin',(-0.00225,-0.01,-0.0076));
#8061=CARTESIAN_POINT('Origin',(-0.02125,-0.01625,-0.01));
#8062=CARTESIAN_POINT('Origin',(-0.02125,-0.01,-0.0076));
#8063=CARTESIAN_POINT('Origin',(-0.01825,-0.01625,-0.01));
#8064=CARTESIAN_POINT('Origin',(-0.01825,-0.01,-0.0076));
#8065=CARTESIAN_POINT('Origin',(0.,0.,-0.01));
#8066=CARTESIAN_POINT('',(-0.02675,-0.00278889744907202,-0.01));
#8067=CARTESIAN_POINT('',(-0.02675,-0.00278889744907202,-0.01));
#8068=CARTESIAN_POINT('',(-0.02675,-0.00278889744907202,-0.01));
#8069=CARTESIAN_POINT('',(-0.02675,-0.00278889744907202,-0.01));
#8070=CARTESIAN_POINT('',(-0.02675,-0.00278889744907202,-0.01));
#8071=CARTESIAN_POINT('Origin',(-0.02675,-0.01,-0.0076));
#8072=CARTESIAN_POINT('',(0.01825,-0.0025,-0.00637117942725555));
#8073=CARTESIAN_POINT('',(0.01825,-0.00792727272727273,-0.000288105467603312));
#8074=CARTESIAN_POINT('Origin',(0.01825,-0.01,-0.0076));
#8075=CARTESIAN_POINT('',(0.02125,-0.00792727272727273,-0.000288105467603312));
#8076=CARTESIAN_POINT('',(-0.02675,-0.00792727272727273,-0.000288105467603312));
#8077=CARTESIAN_POINT('',(0.02125,-0.0025,-0.00637117942725555));
#8078=CARTESIAN_POINT('Origin',(0.02125,-0.01,-0.0076));
#8079=CARTESIAN_POINT('',(-0.02675,-0.0025,-0.00637117942725555));
#8080=CARTESIAN_POINT('',(0.00225,-0.0025,-0.0063711794272556));
#8081=CARTESIAN_POINT('',(0.00225,-0.00792727272727272,-0.000288105467603314));
#8082=CARTESIAN_POINT('Origin',(0.00225,-0.01,-0.0076));
#8083=CARTESIAN_POINT('',(0.00525,-0.00792727272727272,-0.000288105467603314));
#8084=CARTESIAN_POINT('',(-0.02675,-0.00792727272727272,-0.000288105467603312));
#8085=CARTESIAN_POINT('',(0.00525,-0.0025,-0.0063711794272556));
#8086=CARTESIAN_POINT('Origin',(0.00525,-0.01,-0.0076));
#8087=CARTESIAN_POINT('',(-0.02675,-0.0025,-0.0063711794272556));
#8088=CARTESIAN_POINT('',(0.02125,-0.0120727272727273,-0.000288105467603312));
#8089=CARTESIAN_POINT('',(0.01825,-0.0120727272727273,-0.000288105467603312));
#8090=CARTESIAN_POINT('',(-0.02675,-0.0120727272727273,-0.00028810546760331));
#8091=CARTESIAN_POINT('',(0.01825,-0.0175,-0.00637117942725553));
#8092=CARTESIAN_POINT('Origin',(0.01825,-0.01,-0.0076));
#8093=CARTESIAN_POINT('',(0.02125,-0.0175,-0.00637117942725553));
#8094=CARTESIAN_POINT('',(-0.02675,-0.0175,-0.00637117942725553));
#8095=CARTESIAN_POINT('Origin',(0.02125,-0.01,-0.0076));
#8096=CARTESIAN_POINT('',(0.00525,-0.0120727272727273,-0.000288105467603312));
#8097=CARTESIAN_POINT('',(0.00225,-0.0120727272727273,-0.000288105467603312));
#8098=CARTESIAN_POINT('',(-0.02675,-0.0120727272727273,-0.00028810546760331));
#8099=CARTESIAN_POINT('',(0.00225,-0.0175,-0.00637117942725553));
#8100=CARTESIAN_POINT('Origin',(0.00225,-0.01,-0.0076));
#8101=CARTESIAN_POINT('',(0.00525,-0.0175,-0.00637117942725553));
#8102=CARTESIAN_POINT('',(-0.02675,-0.0175,-0.00637117942725553));
#8103=CARTESIAN_POINT('Origin',(0.00525,-0.01,-0.0076));
#8104=CARTESIAN_POINT('',(-0.00525,-0.00792727272727272,-0.000288105467603314));
#8105=CARTESIAN_POINT('',(-0.00225,-0.00792727272727272,-0.000288105467603314));
#8106=CARTESIAN_POINT('',(-0.02675,-0.00792727272727272,-0.000288105467603312));
#8107=CARTESIAN_POINT('',(-0.00225,-0.0025,-0.00637117942725556));
#8108=CARTESIAN_POINT('Origin',(-0.00225,-0.01,-0.0076));
#8109=CARTESIAN_POINT('',(-0.00525,-0.0025,-0.00637117942725555));
#8110=CARTESIAN_POINT('',(-0.02675,-0.0025,-0.00637117942725556));
#8111=CARTESIAN_POINT('Origin',(-0.00525,-0.01,-0.0076));
#8112=CARTESIAN_POINT('',(-0.00225,-0.0120727272727273,-0.000288105467603309));
#8113=CARTESIAN_POINT('',(-0.00525,-0.0120727272727273,-0.000288105467603309));
#8114=CARTESIAN_POINT('',(-0.02675,-0.0120727272727273,-0.000288105467603309));
#8115=CARTESIAN_POINT('',(-0.00525,-0.0175,-0.00637117942725553));
#8116=CARTESIAN_POINT('Origin',(-0.00525,-0.01,-0.0076));
#8117=CARTESIAN_POINT('',(-0.00225,-0.0175,-0.00637117942725553));
#8118=CARTESIAN_POINT('',(-0.02675,-0.0175,-0.00637117942725553));
#8119=CARTESIAN_POINT('Origin',(-0.00225,-0.01,-0.0076));
#8120=CARTESIAN_POINT('',(-0.02125,-0.0025,-0.00637117942725555));
#8121=CARTESIAN_POINT('',(-0.02125,-0.00792727272727273,-0.000288105467603312));
#8122=CARTESIAN_POINT('Origin',(-0.02125,-0.01,-0.0076));
#8123=CARTESIAN_POINT('',(-0.01825,-0.00792727272727273,-0.000288105467603312));
#8124=CARTESIAN_POINT('',(-0.02675,-0.00792727272727273,-0.000288105467603312));
#8125=CARTESIAN_POINT('',(-0.01825,-0.0025,-0.00637117942725555));
#8126=CARTESIAN_POINT('Origin',(-0.01825,-0.01,-0.0076));
#8127=CARTESIAN_POINT('',(-0.02675,-0.0025,-0.00637117942725555));
#8128=CARTESIAN_POINT('',(-0.01825,-0.0120727272727273,-0.000288105467603312));
#8129=CARTESIAN_POINT('',(-0.02125,-0.0120727272727273,-0.000288105467603312));
#8130=CARTESIAN_POINT('',(-0.02675,-0.0120727272727273,-0.00028810546760331));
#8131=CARTESIAN_POINT('',(-0.02125,-0.0175,-0.00637117942725553));
#8132=CARTESIAN_POINT('Origin',(-0.02125,-0.01,-0.0076));
#8133=CARTESIAN_POINT('',(-0.01825,-0.0175,-0.00637117942725553));
#8134=CARTESIAN_POINT('',(-0.02675,-0.0175,-0.00637117942725553));
#8135=CARTESIAN_POINT('Origin',(-0.01825,-0.01,-0.0076));
#8136=CARTESIAN_POINT('Origin',(-0.01825,-0.01625,-0.01));
#8137=CARTESIAN_POINT('',(-0.01825,-0.0147131249905032,0.000812352359916264));
#8138=CARTESIAN_POINT('Origin',(-0.01825,-0.0127,-0.0003));
#8139=CARTESIAN_POINT('Origin',(-0.01825,-0.0127,0.00192470471983253));
#8140=CARTESIAN_POINT('',(-0.01825,-0.0175,-0.01));
#8141=CARTESIAN_POINT('Origin',(-0.01975,-0.0175,-0.01));
#8142=CARTESIAN_POINT('',(-0.02125,-0.0175,-0.01));
#8143=CARTESIAN_POINT('Origin',(-0.02125,-0.01625,-0.01));
#8144=CARTESIAN_POINT('',(-0.02125,-0.0147131249905032,0.000812352359916264));
#8145=CARTESIAN_POINT('Origin',(-0.02125,-0.0127,0.00192470471983253));
#8146=CARTESIAN_POINT('Origin',(-0.02125,-0.0127,-0.0003));
#8147=CARTESIAN_POINT('Origin',(-0.01975,-0.0025,-0.01));
#8148=CARTESIAN_POINT('',(-0.01825,-0.0025,-0.01));
#8149=CARTESIAN_POINT('',(-0.02125,-0.0025,-0.01));
#8150=CARTESIAN_POINT('Origin',(-0.01825,-0.00375,-0.01));
#8151=CARTESIAN_POINT('',(-0.01825,-0.00528687500949675,0.000812352359916264));
#8152=CARTESIAN_POINT('Origin',(-0.01825,-0.0073,0.00192470471983253));
#8153=CARTESIAN_POINT('Origin',(-0.01825,-0.0073,-0.0003));
#8154=CARTESIAN_POINT('Origin',(-0.02125,-0.00375,-0.01));
#8155=CARTESIAN_POINT('',(-0.02125,-0.00528687500949675,0.000812352359916264));
#8156=CARTESIAN_POINT('Origin',(-0.02125,-0.0073,-0.0003));
#8157=CARTESIAN_POINT('Origin',(-0.02125,-0.0073,0.00192470471983253));
#8158=CARTESIAN_POINT('Origin',(-0.00225,-0.01625,-0.01));
#8159=CARTESIAN_POINT('',(-0.00225,-0.0147131249905032,0.000812352359916279));
#8160=CARTESIAN_POINT('Origin',(-0.00225,-0.0127,-0.0003));
#8161=CARTESIAN_POINT('Origin',(-0.00225,-0.0127,0.00192470471983253));
#8162=CARTESIAN_POINT('',(-0.00225,-0.0175,-0.01));
#8163=CARTESIAN_POINT('Origin',(-0.00375,-0.0175,-0.01));
#8164=CARTESIAN_POINT('',(-0.00525,-0.0175,-0.01));
#8165=CARTESIAN_POINT('Origin',(-0.00525,-0.01625,-0.01));
#8166=CARTESIAN_POINT('',(-0.00525,-0.0147131249905032,0.000812352359916277));
#8167=CARTESIAN_POINT('Origin',(-0.00525,-0.0127,0.00192470471983253));
#8168=CARTESIAN_POINT('Origin',(-0.00525,-0.0127,-0.0003));
#8169=CARTESIAN_POINT('Origin',(-0.00525,-0.00375,-0.01));
#8170=CARTESIAN_POINT('',(-0.00525,-0.00528687500949675,0.000812352359916257));
#8171=CARTESIAN_POINT('Origin',(-0.00525,-0.0073,-0.0003));
#8172=CARTESIAN_POINT('Origin',(-0.00525,-0.0073,0.00192470471983252));
#8173=CARTESIAN_POINT('',(-0.00525,-0.0025,-0.01));
#8174=CARTESIAN_POINT('Origin',(-0.00375,-0.0025,-0.01));
#8175=CARTESIAN_POINT('',(-0.00225,-0.0025,-0.01));
#8176=CARTESIAN_POINT('Origin',(-0.00225,-0.00375,-0.01));
#8177=CARTESIAN_POINT('',(-0.00225,-0.00528687500949675,0.000812352359916256));
#8178=CARTESIAN_POINT('Origin',(-0.00225,-0.0073,0.00192470471983252));
#8179=CARTESIAN_POINT('Origin',(-0.00225,-0.0073,-0.0003));
#8180=CARTESIAN_POINT('Origin',(0.00525,-0.01625,-0.01));
#8181=CARTESIAN_POINT('',(0.00525,-0.0147131249905032,0.000812352359916264));
#8182=CARTESIAN_POINT('Origin',(0.00525,-0.0127,-0.0003));
#8183=CARTESIAN_POINT('Origin',(0.00525,-0.0127,0.00192470471983253));
#8184=CARTESIAN_POINT('',(0.00525,-0.0175,-0.01));
#8185=CARTESIAN_POINT('Origin',(0.00375,-0.0175,-0.01));
#8186=CARTESIAN_POINT('',(0.00225,-0.0175,-0.01));
#8187=CARTESIAN_POINT('Origin',(0.00225,-0.01625,-0.01));
#8188=CARTESIAN_POINT('',(0.00225,-0.0147131249905032,0.000812352359916264));
#8189=CARTESIAN_POINT('Origin',(0.00225,-0.0127,0.00192470471983253));
#8190=CARTESIAN_POINT('Origin',(0.00225,-0.0127,-0.0003));
#8191=CARTESIAN_POINT('Origin',(0.02125,-0.01625,-0.01));
#8192=CARTESIAN_POINT('',(0.02125,-0.0147131249905032,0.000812352359916264));
#8193=CARTESIAN_POINT('Origin',(0.02125,-0.0127,-0.0003));
#8194=CARTESIAN_POINT('Origin',(0.02125,-0.0127,0.00192470471983253));
#8195=CARTESIAN_POINT('',(0.02125,-0.0175,-0.01));
#8196=CARTESIAN_POINT('Origin',(0.01975,-0.0175,-0.01));
#8197=CARTESIAN_POINT('',(0.01825,-0.0175,-0.01));
#8198=CARTESIAN_POINT('Origin',(0.01825,-0.01625,-0.01));
#8199=CARTESIAN_POINT('',(0.01825,-0.0147131249905032,0.000812352359916264));
#8200=CARTESIAN_POINT('Origin',(0.01825,-0.0127,0.00192470471983253));
#8201=CARTESIAN_POINT('Origin',(0.01825,-0.0127,-0.0003));
#8202=CARTESIAN_POINT('Origin',(0.00375,-0.0025,-0.01));
#8203=CARTESIAN_POINT('',(0.00525,-0.0025,-0.01));
#8204=CARTESIAN_POINT('',(0.00225,-0.0025,-0.01));
#8205=CARTESIAN_POINT('Origin',(0.00525,-0.00375,-0.01));
#8206=CARTESIAN_POINT('',(0.00525,-0.00528687500949675,0.000812352359916255));
#8207=CARTESIAN_POINT('Origin',(0.00525,-0.0073,0.00192470471983252));
#8208=CARTESIAN_POINT('Origin',(0.00525,-0.0073,-0.0003));
#8209=CARTESIAN_POINT('Origin',(0.00225,-0.00375,-0.01));
#8210=CARTESIAN_POINT('',(0.00225,-0.00528687500949675,0.000812352359916255));
#8211=CARTESIAN_POINT('Origin',(0.00225,-0.0073,-0.0003));
#8212=CARTESIAN_POINT('Origin',(0.00225,-0.0073,0.00192470471983252));
#8213=CARTESIAN_POINT('Origin',(0.01975,-0.0025,-0.01));
#8214=CARTESIAN_POINT('',(0.02125,-0.0025,-0.01));
#8215=CARTESIAN_POINT('',(0.01825,-0.0025,-0.01));
#8216=CARTESIAN_POINT('Origin',(0.02125,-0.00375,-0.01));
#8217=CARTESIAN_POINT('',(0.02125,-0.00528687500949675,0.000812352359916264));
#8218=CARTESIAN_POINT('Origin',(0.02125,-0.0073,0.00192470471983253));
#8219=CARTESIAN_POINT('Origin',(0.02125,-0.0073,-0.0003));
#8220=CARTESIAN_POINT('Origin',(0.01825,-0.00375,-0.01));
#8221=CARTESIAN_POINT('',(0.01825,-0.00528687500949675,0.000812352359916264));
#8222=CARTESIAN_POINT('Origin',(0.01825,-0.0073,-0.0003));
#8223=CARTESIAN_POINT('Origin',(0.01825,-0.0073,0.00192470471983253));
#8224=CARTESIAN_POINT('Origin',(-0.02675,-0.0127,0.00192470471983253));
#8225=CARTESIAN_POINT('',(-0.00375,-0.0147131249905032,0.000812352359916278));
#8226=CARTESIAN_POINT('Origin',(-0.00375,-0.0127,-0.0003));
#8227=CARTESIAN_POINT('Origin',(-0.02675,-0.0127,0.00192470471983253));
#8228=CARTESIAN_POINT('',(0.00375,-0.0147131249905032,0.000812352359916264));
#8229=CARTESIAN_POINT('Origin',(0.00375,-0.0127,-0.0003));
#8230=CARTESIAN_POINT('Origin',(-0.02675,-0.0127,0.00192470471983253));
#8231=CARTESIAN_POINT('',(0.01975,-0.0147131249905032,0.000812352359916264));
#8232=CARTESIAN_POINT('Origin',(0.01975,-0.0127,-0.0003));
#8233=CARTESIAN_POINT('Origin',(-0.02675,-0.0073,0.00192470471983253));
#8234=CARTESIAN_POINT('',(0.01975,-0.00528687500949675,0.000812352359916264));
#8235=CARTESIAN_POINT('Origin',(0.,-0.0073,-0.0003));
#8236=CARTESIAN_POINT('Origin',(-0.02675,-0.0073,0.00192470471983252));
#8237=CARTESIAN_POINT('',(0.00375,-0.00528687500949675,0.000812352359916255));
#8238=CARTESIAN_POINT('Origin',(-2.11058022910511E-18,-0.0073,-0.0003));
#8239=CARTESIAN_POINT('Origin',(-0.02675,-0.0073,0.00192470471983252));
#8240=CARTESIAN_POINT('',(-0.00375,-0.00528687500949675,0.000812352359916257));
#8241=CARTESIAN_POINT('Origin',(-0.00375,-0.0073,-0.0003));
#8242=CARTESIAN_POINT('Origin',(-0.02675,-0.0073,0.00192470471983253));
#8243=CARTESIAN_POINT('',(-0.01975,-0.00528687500949675,0.000812352359916264));
#8244=CARTESIAN_POINT('Origin',(0.,-0.0073,-0.0003));
#8245=CARTESIAN_POINT('Origin',(-0.02675,-0.0127,0.00192470471983253));
#8246=CARTESIAN_POINT('',(-0.01975,-0.0147131249905032,0.000812352359916264));
#8247=CARTESIAN_POINT('Origin',(-0.01975,-0.0127,-0.0003));
#8248=CARTESIAN_POINT('Origin',(0.01825,-0.00375,0.061));
#8249=CARTESIAN_POINT('',(0.01825,-0.0025,0.0598288205727444));
#8250=CARTESIAN_POINT('',(0.01825,-0.00278889744907202,0.061));
#8251=CARTESIAN_POINT('Origin',(0.01825,-0.01,0.0586));
#8252=CARTESIAN_POINT('',(0.01825,-0.0025,0.061));
#8253=CARTESIAN_POINT('',(0.01825,-0.0025,0.061));
#8254=CARTESIAN_POINT('',(0.01825,-0.00375,0.061));
#8255=CARTESIAN_POINT('Origin',(0.01975,-0.0025,0.061));
#8256=CARTESIAN_POINT('',(0.02125,-0.0025,0.0598288205727444));
#8257=CARTESIAN_POINT('',(0.02675,-0.0025,0.0598288205727444));
#8258=CARTESIAN_POINT('',(0.02125,-0.0025,0.061));
#8259=CARTESIAN_POINT('',(0.02125,-0.0025,0.061));
#8260=CARTESIAN_POINT('',(0.01975,-0.0025,0.061));
#8261=CARTESIAN_POINT('Origin',(0.02125,-0.00375,0.061));
#8262=CARTESIAN_POINT('',(0.02125,-0.00278889744907202,0.061));
#8263=CARTESIAN_POINT('Origin',(0.02125,-0.01,0.0586));
#8264=CARTESIAN_POINT('',(0.02125,-0.00375,0.061));
#8265=CARTESIAN_POINT('Origin',(0.00375,-0.0025,0.061));
#8266=CARTESIAN_POINT('',(0.00525,-0.0025,0.0598288205727444));
#8267=CARTESIAN_POINT('',(0.02675,-0.0025,0.0598288205727444));
#8268=CARTESIAN_POINT('',(0.00525,-0.0025,0.061));
#8269=CARTESIAN_POINT('',(0.00525,-0.0025,0.061));
#8270=CARTESIAN_POINT('',(0.00375,-0.0025,0.061));
#8271=CARTESIAN_POINT('Origin',(0.00525,-0.00375,0.061));
#8272=CARTESIAN_POINT('',(0.00525,-0.00278889744907202,0.061));
#8273=CARTESIAN_POINT('Origin',(0.00525,-0.01,0.0586));
#8274=CARTESIAN_POINT('',(0.00525,-0.00375,0.061));
#8275=CARTESIAN_POINT('Origin',(-0.00525,-0.01625,0.061));
#8276=CARTESIAN_POINT('Origin',(-0.00525,-0.01,0.0586));
#8277=CARTESIAN_POINT('Origin',(-0.00525,-0.00375,0.061));
#8278=CARTESIAN_POINT('',(-0.00525,-0.0025,0.0598288205727444));
#8279=CARTESIAN_POINT('',(-0.00525,-0.00278889744907202,0.061));
#8280=CARTESIAN_POINT('Origin',(-0.00525,-0.01,0.0586));
#8281=CARTESIAN_POINT('',(-0.00525,-0.0025,0.061));
#8282=CARTESIAN_POINT('',(-0.00525,-0.0025,0.061));
#8283=CARTESIAN_POINT('',(-0.00525,-0.00375,0.061));
#8284=CARTESIAN_POINT('Origin',(-0.00375,-0.0025,0.061));
#8285=CARTESIAN_POINT('',(0.02675,-0.0025,0.0598288205727444));
#8286=CARTESIAN_POINT('',(-0.00375,-0.0025,0.061));
#8287=CARTESIAN_POINT('Origin',(-0.02125,-0.00375,0.061));
#8288=CARTESIAN_POINT('',(-0.02125,-0.0025,0.0598288205727444));
#8289=CARTESIAN_POINT('',(-0.02125,-0.00278889744907202,0.061));
#8290=CARTESIAN_POINT('Origin',(-0.02125,-0.01,0.0586));
#8291=CARTESIAN_POINT('',(-0.02125,-0.0025,0.061));
#8292=CARTESIAN_POINT('',(-0.02125,-0.0025,0.061));
#8293=CARTESIAN_POINT('',(-0.02125,-0.00375,0.061));
#8294=CARTESIAN_POINT('Origin',(-0.01975,-0.0025,0.061));
#8295=CARTESIAN_POINT('',(-0.01825,-0.0025,0.0598288205727444));
#8296=CARTESIAN_POINT('',(0.02675,-0.0025,0.0598288205727444));
#8297=CARTESIAN_POINT('',(-0.01825,-0.0025,0.061));
#8298=CARTESIAN_POINT('',(-0.01825,-0.0025,0.061));
#8299=CARTESIAN_POINT('',(-0.01975,-0.0025,0.061));
#8300=CARTESIAN_POINT('Origin',(-0.01825,-0.00375,0.061));
#8301=CARTESIAN_POINT('',(-0.01825,-0.00278889744907202,0.061));
#8302=CARTESIAN_POINT('Origin',(-0.01825,-0.01,0.0586));
#8303=CARTESIAN_POINT('',(-0.01825,-0.00375,0.061));
#8304=CARTESIAN_POINT('Origin',(0.00375,-0.0175,0.061));
#8305=CARTESIAN_POINT('',(0.02675,-0.0175,0.0598288205727445));
#8306=CARTESIAN_POINT('Origin',(-0.01975,-0.0175,0.061));
#8307=CARTESIAN_POINT('',(0.02675,-0.0175,0.0598288205727445));
#8308=CARTESIAN_POINT('Origin',(0.01975,-0.0175,0.061));
#8309=CARTESIAN_POINT('',(0.02675,-0.0175,0.0598288205727445));
#8310=CARTESIAN_POINT('Origin',(-3.46944695195361E-18,0.,0.061));
#8311=CARTESIAN_POINT('',(0.02675,-0.00278889744907202,0.061));
#8312=CARTESIAN_POINT('',(0.02675,-0.00278889744907202,0.061));
#8313=CARTESIAN_POINT('',(0.02675,-0.00278889744907202,0.061));
#8314=CARTESIAN_POINT('',(0.02675,-0.00278889744907202,0.061));
#8315=CARTESIAN_POINT('',(0.02675,-0.00278889744907202,0.061));
#8316=CARTESIAN_POINT('Origin',(0.02675,-0.01,0.0586));
#8317=CARTESIAN_POINT('',(0.00225,-0.0175,0.0573711794272556));
#8318=CARTESIAN_POINT('',(0.00225,-0.0120727272727273,0.0512881054676033));
#8319=CARTESIAN_POINT('Origin',(0.00225,-0.01,0.0586));
#8320=CARTESIAN_POINT('',(0.00525,-0.0120727272727273,0.0512881054676033));
#8321=CARTESIAN_POINT('',(0.02675,-0.0120727272727273,0.0512881054676033));
#8322=CARTESIAN_POINT('',(0.00525,-0.0175,0.0573711794272556));
#8323=CARTESIAN_POINT('Origin',(0.00525,-0.01,0.0586));
#8324=CARTESIAN_POINT('',(0.02675,-0.0175,0.0573711794272556));
#8325=CARTESIAN_POINT('',(0.02125,-0.00792727272727272,0.0512881054676033));
#8326=CARTESIAN_POINT('',(0.01825,-0.00792727272727272,0.0512881054676033));
#8327=CARTESIAN_POINT('',(0.02675,-0.00792727272727272,0.0512881054676033));
#8328=CARTESIAN_POINT('',(0.01825,-0.0025,0.0573711794272556));
#8329=CARTESIAN_POINT('Origin',(0.01825,-0.01,0.0586));
#8330=CARTESIAN_POINT('',(0.02125,-0.0025,0.0573711794272556));
#8331=CARTESIAN_POINT('',(0.02675,-0.0025,0.0573711794272556));
#8332=CARTESIAN_POINT('Origin',(0.02125,-0.01,0.0586));
#8333=CARTESIAN_POINT('',(0.00525,-0.00792727272727272,0.0512881054676033));
#8334=CARTESIAN_POINT('',(0.00225,-0.00792727272727272,0.0512881054676033));
#8335=CARTESIAN_POINT('',(0.02675,-0.00792727272727272,0.0512881054676033));
#8336=CARTESIAN_POINT('',(0.00225,-0.0025,0.0573711794272556));
#8337=CARTESIAN_POINT('Origin',(0.00225,-0.01,0.0586));
#8338=CARTESIAN_POINT('',(0.00525,-0.0025,0.0573711794272556));
#8339=CARTESIAN_POINT('',(0.02675,-0.0025,0.0573711794272556));
#8340=CARTESIAN_POINT('Origin',(0.00525,-0.01,0.0586));
#8341=CARTESIAN_POINT('',(-0.00525,-0.0120727272727273,0.0512881054676033));
#8342=CARTESIAN_POINT('',(-0.00225,-0.0120727272727273,0.0512881054676033));
#8343=CARTESIAN_POINT('',(0.02675,-0.0120727272727273,0.0512881054676033));
#8344=CARTESIAN_POINT('',(-0.00225,-0.0175,0.0573711794272556));
#8345=CARTESIAN_POINT('Origin',(-0.00225,-0.01,0.0586));
#8346=CARTESIAN_POINT('',(-0.00525,-0.0175,0.0573711794272556));
#8347=CARTESIAN_POINT('',(0.02675,-0.0175,0.0573711794272556));
#8348=CARTESIAN_POINT('Origin',(-0.00525,-0.01,0.0586));
#8349=CARTESIAN_POINT('',(-0.00225,-0.00792727272727272,0.0512881054676033));
#8350=CARTESIAN_POINT('',(-0.00525,-0.00792727272727272,0.0512881054676033));
#8351=CARTESIAN_POINT('',(0.02675,-0.00792727272727272,0.0512881054676033));
#8352=CARTESIAN_POINT('',(-0.00525,-0.0025,0.0573711794272556));
#8353=CARTESIAN_POINT('Origin',(-0.00525,-0.01,0.0586));
#8354=CARTESIAN_POINT('',(-0.00225,-0.0025,0.0573711794272556));
#8355=CARTESIAN_POINT('',(0.02675,-0.0025,0.0573711794272556));
#8356=CARTESIAN_POINT('Origin',(-0.00225,-0.01,0.0586));
#8357=CARTESIAN_POINT('',(-0.02125,-0.0175,0.0573711794272556));
#8358=CARTESIAN_POINT('',(-0.02125,-0.0120727272727273,0.0512881054676033));
#8359=CARTESIAN_POINT('Origin',(-0.02125,-0.01,0.0586));
#8360=CARTESIAN_POINT('',(-0.01825,-0.0120727272727273,0.0512881054676033));
#8361=CARTESIAN_POINT('',(0.02675,-0.0120727272727273,0.0512881054676033));
#8362=CARTESIAN_POINT('',(-0.01825,-0.0175,0.0573711794272556));
#8363=CARTESIAN_POINT('Origin',(-0.01825,-0.01,0.0586));
#8364=CARTESIAN_POINT('',(0.02675,-0.0175,0.0573711794272556));
#8365=CARTESIAN_POINT('',(-0.01825,-0.00792727272727272,0.0512881054676033));
#8366=CARTESIAN_POINT('',(-0.02125,-0.00792727272727272,0.0512881054676033));
#8367=CARTESIAN_POINT('',(0.02675,-0.00792727272727272,0.0512881054676033));
#8368=CARTESIAN_POINT('',(-0.02125,-0.0025,0.0573711794272556));
#8369=CARTESIAN_POINT('Origin',(-0.02125,-0.01,0.0586));
#8370=CARTESIAN_POINT('',(-0.01825,-0.0025,0.0573711794272556));
#8371=CARTESIAN_POINT('',(0.02675,-0.0025,0.0573711794272556));
#8372=CARTESIAN_POINT('Origin',(-0.01825,-0.01,0.0586));
#8373=CARTESIAN_POINT('',(0.01825,-0.0175,0.0573711794272556));
#8374=CARTESIAN_POINT('',(0.01825,-0.0120727272727273,0.0512881054676033));
#8375=CARTESIAN_POINT('Origin',(0.01825,-0.01,0.0586));
#8376=CARTESIAN_POINT('',(0.02125,-0.0120727272727273,0.0512881054676033));
#8377=CARTESIAN_POINT('',(0.02675,-0.0120727272727273,0.0512881054676033));
#8378=CARTESIAN_POINT('',(0.02125,-0.0175,0.0573711794272556));
#8379=CARTESIAN_POINT('Origin',(0.02125,-0.01,0.0586));
#8380=CARTESIAN_POINT('',(0.02675,-0.0175,0.0573711794272556));
#8381=CARTESIAN_POINT('Origin',(0.01975,-0.0175,0.061));
#8382=CARTESIAN_POINT('',(0.02125,-0.0175,0.061));
#8383=CARTESIAN_POINT('',(0.01825,-0.0175,0.061));
#8384=CARTESIAN_POINT('Origin',(0.02125,-0.01625,0.061));
#8385=CARTESIAN_POINT('',(0.02125,-0.015,0.0490752952801675));
#8386=CARTESIAN_POINT('Origin',(0.02125,-0.0127,0.0490752952801675));
#8387=CARTESIAN_POINT('',(0.02125,-0.015,0.0483));
#8388=CARTESIAN_POINT('',(0.02125,-0.015,0.061));
#8389=CARTESIAN_POINT('Origin',(0.02125,-0.0127,0.0483));
#8390=CARTESIAN_POINT('Origin',(0.01975,-0.015,0.061));
#8391=CARTESIAN_POINT('',(0.01825,-0.015,0.0490752952801675));
#8392=CARTESIAN_POINT('',(0.01825,-0.015,0.0483));
#8393=CARTESIAN_POINT('',(0.01825,-0.015,0.061));
#8394=CARTESIAN_POINT('',(0.01975,-0.015,0.0483));
#8395=CARTESIAN_POINT('',(0.01975,-0.015,0.0490752952801675));
#8396=CARTESIAN_POINT('Origin',(0.01825,-0.01625,0.061));
#8397=CARTESIAN_POINT('Origin',(0.01825,-0.0127,0.0483));
#8398=CARTESIAN_POINT('Origin',(0.01825,-0.0127,0.0490752952801675));
#8399=CARTESIAN_POINT('Origin',(-0.01975,-0.005,0.061));
#8400=CARTESIAN_POINT('',(-0.01825,-0.005,0.0490752952801675));
#8401=CARTESIAN_POINT('',(-0.01825,-0.005,0.0483));
#8402=CARTESIAN_POINT('',(-0.01825,-0.005,0.061));
#8403=CARTESIAN_POINT('',(-0.02125,-0.005,0.0483));
#8404=CARTESIAN_POINT('',(-0.02125,-0.005,0.0483));
#8405=CARTESIAN_POINT('',(-0.02125,-0.005,0.0490752952801675));
#8406=CARTESIAN_POINT('',(-0.02125,-0.005,0.061));
#8407=CARTESIAN_POINT('',(-0.01825,-0.005,0.0490752952801675));
#8408=CARTESIAN_POINT('Origin',(-0.01825,-0.00375,0.061));
#8409=CARTESIAN_POINT('Origin',(-0.01825,-0.0073,0.0490752952801675));
#8410=CARTESIAN_POINT('',(-0.01825,-0.0025,0.061));
#8411=CARTESIAN_POINT('Origin',(-0.01825,-0.0073,0.0483));
#8412=CARTESIAN_POINT('Origin',(-0.01975,-0.0025,0.061));
#8413=CARTESIAN_POINT('',(-0.02125,-0.0025,0.061));
#8414=CARTESIAN_POINT('Origin',(-0.02125,-0.00375,0.061));
#8415=CARTESIAN_POINT('Origin',(-0.02125,-0.0073,0.0490752952801675));
#8416=CARTESIAN_POINT('Origin',(-0.02125,-0.0073,0.0483));
#8417=CARTESIAN_POINT('Origin',(-0.01975,-0.0175,0.061));
#8418=CARTESIAN_POINT('',(-0.01825,-0.0175,0.061));
#8419=CARTESIAN_POINT('',(-0.02125,-0.0175,0.061));
#8420=CARTESIAN_POINT('Origin',(-0.01825,-0.01625,0.061));
#8421=CARTESIAN_POINT('',(-0.01825,-0.015,0.0490752952801675));
#8422=CARTESIAN_POINT('Origin',(-0.01825,-0.0127,0.0490752952801675));
#8423=CARTESIAN_POINT('',(-0.01825,-0.015,0.0483));
#8424=CARTESIAN_POINT('',(-0.01825,-0.015,0.061));
#8425=CARTESIAN_POINT('Origin',(-0.01825,-0.0127,0.0483));
#8426=CARTESIAN_POINT('Origin',(-0.01975,-0.015,0.061));
#8427=CARTESIAN_POINT('',(-0.02125,-0.015,0.0490752952801675));
#8428=CARTESIAN_POINT('',(-0.02125,-0.015,0.0483));
#8429=CARTESIAN_POINT('',(-0.02125,-0.015,0.061));
#8430=CARTESIAN_POINT('',(-0.01975,-0.015,0.0483));
#8431=CARTESIAN_POINT('',(-0.01975,-0.015,0.0490752952801675));
#8432=CARTESIAN_POINT('Origin',(-0.02125,-0.01625,0.061));
#8433=CARTESIAN_POINT('Origin',(-0.02125,-0.0127,0.0483));
#8434=CARTESIAN_POINT('Origin',(-0.02125,-0.0127,0.0490752952801675));
#8435=CARTESIAN_POINT('Origin',(-0.00375,-0.005,0.061));
#8436=CARTESIAN_POINT('',(-0.00225,-0.005,0.0490752952801675));
#8437=CARTESIAN_POINT('',(-0.00225,-0.005,0.0483));
#8438=CARTESIAN_POINT('',(-0.00225,-0.005,0.061));
#8439=CARTESIAN_POINT('',(-0.00525,-0.005,0.0483));
#8440=CARTESIAN_POINT('',(-0.00525,-0.005,0.0483));
#8441=CARTESIAN_POINT('',(-0.00525,-0.005,0.0490752952801675));
#8442=CARTESIAN_POINT('',(-0.00525,-0.005,0.061));
#8443=CARTESIAN_POINT('',(-0.00225,-0.005,0.0490752952801675));
#8444=CARTESIAN_POINT('Origin',(-0.00225,-0.00375,0.061));
#8445=CARTESIAN_POINT('Origin',(-0.00225,-0.0073,0.0490752952801675));
#8446=CARTESIAN_POINT('',(-0.00225,-0.0025,0.061));
#8447=CARTESIAN_POINT('Origin',(-0.00225,-0.0073,0.0483));
#8448=CARTESIAN_POINT('Origin',(-0.00375,-0.0025,0.061));
#8449=CARTESIAN_POINT('',(-0.00525,-0.0025,0.061));
#8450=CARTESIAN_POINT('Origin',(-0.00525,-0.00375,0.061));
#8451=CARTESIAN_POINT('Origin',(-0.00525,-0.0073,0.0490752952801675));
#8452=CARTESIAN_POINT('Origin',(-0.00525,-0.0073,0.0483));
#8453=CARTESIAN_POINT('Origin',(-0.00375,-0.015,0.061));
#8454=CARTESIAN_POINT('',(-0.00525,-0.015,0.0490752952801675));
#8455=CARTESIAN_POINT('',(-0.00525,-0.015,0.0483));
#8456=CARTESIAN_POINT('',(-0.00525,-0.015,0.061));
#8457=CARTESIAN_POINT('',(-0.00225,-0.015,0.0483));
#8458=CARTESIAN_POINT('',(-0.00225,-0.015,0.0483));
#8459=CARTESIAN_POINT('',(-0.00225,-0.015,0.0490752952801675));
#8460=CARTESIAN_POINT('',(-0.00225,-0.015,0.061));
#8461=CARTESIAN_POINT('',(-0.00525,-0.015,0.0490752952801675));
#8462=CARTESIAN_POINT('Origin',(-0.00525,-0.01625,0.061));
#8463=CARTESIAN_POINT('Origin',(-0.00525,-0.0127,0.0490752952801675));
#8464=CARTESIAN_POINT('',(-0.00525,-0.0175,0.061));
#8465=CARTESIAN_POINT('Origin',(-0.00525,-0.0127,0.0483));
#8466=CARTESIAN_POINT('Origin',(-0.00375,-0.0175,0.061));
#8467=CARTESIAN_POINT('',(-0.00225,-0.0175,0.061));
#8468=CARTESIAN_POINT('Origin',(-0.00225,-0.01625,0.061));
#8469=CARTESIAN_POINT('Origin',(-0.00225,-0.0127,0.0490752952801675));
#8470=CARTESIAN_POINT('Origin',(-0.00225,-0.0127,0.0483));
#8471=CARTESIAN_POINT('Origin',(0.00375,-0.005,0.061));
#8472=CARTESIAN_POINT('',(0.00525,-0.005,0.0490752952801675));
#8473=CARTESIAN_POINT('',(0.00525,-0.005,0.0483));
#8474=CARTESIAN_POINT('',(0.00525,-0.005,0.061));
#8475=CARTESIAN_POINT('',(0.00225,-0.005,0.0483));
#8476=CARTESIAN_POINT('',(0.00225,-0.005,0.0483));
#8477=CARTESIAN_POINT('',(0.00225,-0.005,0.0490752952801675));
#8478=CARTESIAN_POINT('',(0.00225,-0.005,0.061));
#8479=CARTESIAN_POINT('',(0.00525,-0.005,0.0490752952801675));
#8480=CARTESIAN_POINT('Origin',(0.00525,-0.00375,0.061));
#8481=CARTESIAN_POINT('Origin',(0.00525,-0.0073,0.0490752952801675));
#8482=CARTESIAN_POINT('',(0.00525,-0.0025,0.061));
#8483=CARTESIAN_POINT('Origin',(0.00525,-0.0073,0.0483));
#8484=CARTESIAN_POINT('Origin',(0.00375,-0.0025,0.061));
#8485=CARTESIAN_POINT('',(0.00225,-0.0025,0.061));
#8486=CARTESIAN_POINT('Origin',(0.00225,-0.00375,0.061));
#8487=CARTESIAN_POINT('Origin',(0.00225,-0.0073,0.0490752952801675));
#8488=CARTESIAN_POINT('Origin',(0.00225,-0.0073,0.0483));
#8489=CARTESIAN_POINT('Origin',(0.01975,-0.005,0.061));
#8490=CARTESIAN_POINT('',(0.02125,-0.005,0.0490752952801675));
#8491=CARTESIAN_POINT('',(0.02125,-0.005,0.0483));
#8492=CARTESIAN_POINT('',(0.02125,-0.005,0.061));
#8493=CARTESIAN_POINT('',(0.01825,-0.005,0.0483));
#8494=CARTESIAN_POINT('',(0.01825,-0.005,0.0483));
#8495=CARTESIAN_POINT('',(0.01825,-0.005,0.0490752952801675));
#8496=CARTESIAN_POINT('',(0.01825,-0.005,0.061));
#8497=CARTESIAN_POINT('',(0.02125,-0.005,0.0490752952801675));
#8498=CARTESIAN_POINT('Origin',(0.02125,-0.00375,0.061));
#8499=CARTESIAN_POINT('Origin',(0.02125,-0.0073,0.0490752952801675));
#8500=CARTESIAN_POINT('',(0.02125,-0.0025,0.061));
#8501=CARTESIAN_POINT('Origin',(0.02125,-0.0073,0.0483));
#8502=CARTESIAN_POINT('Origin',(0.01975,-0.0025,0.061));
#8503=CARTESIAN_POINT('',(0.01825,-0.0025,0.061));
#8504=CARTESIAN_POINT('Origin',(0.01825,-0.00375,0.061));
#8505=CARTESIAN_POINT('Origin',(0.01825,-0.0073,0.0490752952801675));
#8506=CARTESIAN_POINT('Origin',(0.01825,-0.0073,0.0483));
#8507=CARTESIAN_POINT('Origin',(0.00375,-0.0175,0.061));
#8508=CARTESIAN_POINT('',(0.00525,-0.0175,0.061));
#8509=CARTESIAN_POINT('',(0.00225,-0.0175,0.061));
#8510=CARTESIAN_POINT('Origin',(0.00525,-0.01625,0.061));
#8511=CARTESIAN_POINT('',(0.00525,-0.015,0.0490752952801675));
#8512=CARTESIAN_POINT('Origin',(0.00525,-0.0127,0.0490752952801675));
#8513=CARTESIAN_POINT('',(0.00525,-0.015,0.0483));
#8514=CARTESIAN_POINT('',(0.00525,-0.015,0.061));
#8515=CARTESIAN_POINT('Origin',(0.00525,-0.0127,0.0483));
#8516=CARTESIAN_POINT('Origin',(0.00375,-0.015,0.061));
#8517=CARTESIAN_POINT('',(0.00225,-0.015,0.0490752952801675));
#8518=CARTESIAN_POINT('',(0.00225,-0.015,0.0483));
#8519=CARTESIAN_POINT('',(0.00225,-0.015,0.061));
#8520=CARTESIAN_POINT('',(0.00375,-0.015,0.0483));
#8521=CARTESIAN_POINT('',(0.00375,-0.015,0.0490752952801675));
#8522=CARTESIAN_POINT('Origin',(0.00225,-0.01625,0.061));
#8523=CARTESIAN_POINT('Origin',(0.00225,-0.0127,0.0483));
#8524=CARTESIAN_POINT('Origin',(0.00225,-0.0127,0.0490752952801675));
#8525=CARTESIAN_POINT('Origin',(-0.01975,-0.0127,0.0483));
#8526=CARTESIAN_POINT('Origin',(0.,-0.0127,0.0483));
#8527=CARTESIAN_POINT('Origin',(0.00375,-0.0127,0.0483));
#8528=CARTESIAN_POINT('Origin',(0.01975,-0.0127,0.0483));
#8529=CARTESIAN_POINT('Origin',(0.,-0.0073,0.0483));
#8530=CARTESIAN_POINT('Origin',(0.,-0.0073,0.0483));
#8531=CARTESIAN_POINT('Origin',(0.,-0.0073,0.0483));
#8532=CARTESIAN_POINT('Origin',(0.,-0.0073,0.0483));
#8533=CARTESIAN_POINT('Origin',(0.02675,-0.0127,0.0490752952801675));
#8534=CARTESIAN_POINT('Origin',(0.02675,-0.0073,0.0490752952801675));
#8535=CARTESIAN_POINT('Origin',(0.02675,-0.0073,0.0490752952801675));
#8536=CARTESIAN_POINT('Origin',(0.02675,-0.0127,0.0490752952801675));
#8537=CARTESIAN_POINT('Origin',(0.02675,-0.0073,0.0490752952801675));
#8538=CARTESIAN_POINT('Origin',(0.02675,-0.0127,0.0490752952801675));
#8539=CARTESIAN_POINT('Origin',(0.02675,-0.0073,0.0490752952801675));
#8540=CARTESIAN_POINT('Origin',(0.02675,-0.0127,0.0490752952801675));
#8541=CARTESIAN_POINT('Origin',(0.,0.005,-0.005));
#8923=UNCERTAINTY_MEASURE_WITH_UNIT(LENGTH_MEASURE(1.E-5),#8945,
'DISTANCE_ACCURACY_VALUE',
'Maximum model space distance between geometric entities at asserted c
onnectivities');
#8932=UNCERTAINTY_MEASURE_WITH_UNIT(LENGTH_MEASURE(1.E-5),#8945,
'DISTANCE_ACCURACY_VALUE',
'Maximum model space distance between geometric entities at asserted c
onnectivities');
#8935=(
GEOMETRIC_REPRESENTATION_CONTEXT(3)
GLOBAL_UNCERTAINTY_ASSIGNED_CONTEXT((#8923))
GLOBAL_UNIT_ASSIGNED_CONTEXT((#8945,#8946,#8947))
REPRESENTATION_CONTEXT('','3D')
);
#8944=(
GEOMETRIC_REPRESENTATION_CONTEXT(3)
GLOBAL_UNCERTAINTY_ASSIGNED_CONTEXT((#8932))
GLOBAL_UNIT_ASSIGNED_CONTEXT((#8945,#8946,#8947))
REPRESENTATION_CONTEXT('','3D')
);
#8945=(
LENGTH_UNIT()
NAMED_UNIT(*)
SI_UNIT($,.METRE.)
);
#8946=(
NAMED_UNIT(*)
PLANE_ANGLE_UNIT()
SI_UNIT($,.RADIAN.)
);
#8947=(
NAMED_UNIT(*)
SI_UNIT($,.STERADIAN.)
SOLID_ANGLE_UNIT()
);
#8950=SHAPE_DEFINITION_REPRESENTATION(#8961,#8994);
#8961=PRODUCT_DEFINITION_SHAPE('',$,#9006);
#8994=SHAPE_REPRESENTATION('',(#5308),#8935);
#9003=PRODUCT_DEFINITION_CONTEXT('part definition',#9038,'design');
#9006=PRODUCT_DEFINITION('Motor Mount','Motor Mount',#9017,#9003);
#9017=PRODUCT_DEFINITION_FORMATION('',$,#9042);
#9038=APPLICATION_CONTEXT('Managed model based 3d engineering');
#9039=PRODUCT_CONTEXT('part definition',#9038,'mechanical');
#9042=PRODUCT('Motor Mount','Motor Mount',
'LEGAL AND USAGE DISCLAIMER: this Data/Model is provided \X2\201C\X0\A
S IS\X2\201D\X0\ for informational and representational only. It is a 
geometric approximation and is NOT engineered, certified, or guarantee
d for dimensional accuracy, exact tolerances, or production-level prec
ision. Vendor disclaims all implied warranties including fitness for a
 particular purpose. DO NOT USE FOR DIRECT PHYSICAL MANUFACTURING, AUT
OMATED PRODUCTION, OR SAFETY-CRITICAL SYSTEMS without independent engi
neering verification and resolution of any design discrepancies.',(#9039));
#9053=PRESENTATION_STYLE_ASSIGNMENT((#9058));
#9058=SURFACE_STYLE_USAGE(.BOTH.,#9063);
#9063=SURFACE_SIDE_STYLE('',(#9068));
#9068=SURFACE_STYLE_FILL_AREA(#9073);
#9073=FILL_AREA_STYLE('Opaque(89,149,218)',(#9078));
#9078=FILL_AREA_STYLE_COLOUR('Opaque(89,149,218)',#9083);
#9083=COLOUR_RGB('Opaque(89,149,218)',0.349019607843137,0.584313725490196,
0.854901960784314);
ENDSEC;
END-ISO-10303-21;
